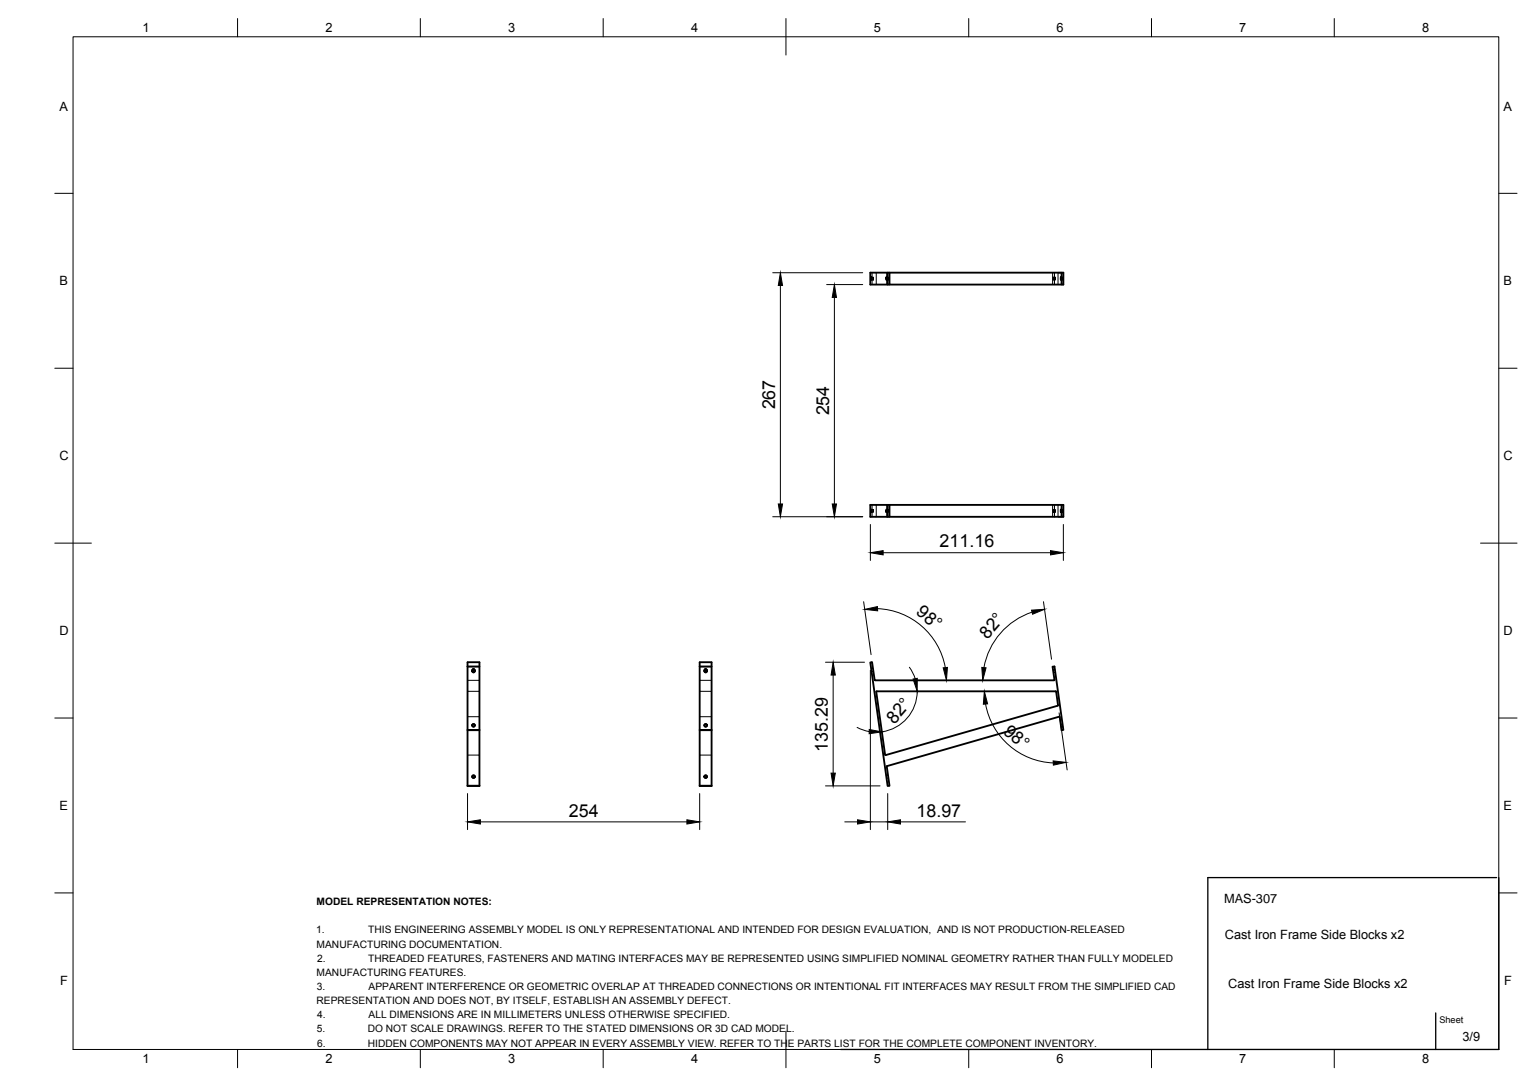
ISO-10303-21;
HEADER;
FILE_DESCRIPTION (('STEP AP214'),
    '1' );
FILE_NAME ('Cast Iron Frame Side Blocks x2.step',
    '2026-10-06T07:34:29',
    ( '' ),
    ( '' ),
    'SwSTEP 2.0',
    'SolidWorks 2025',
    '' );
FILE_SCHEMA (( 'AUTOMOTIVE_DESIGN' ));
ENDSEC;

DATA;
#2=DIRECTION ( 'NONE',  ( 0.000000000000000000, 0.000000000000000000, -1.000000000000000000 ) ) ;
#4=CARTESIAN_POINT ( 'NONE',  ( 177.5000000000000853, 15.47035339324670922, 37.00486596562913633 ) ) ;
#7=CARTESIAN_POINT ( 'NONE',  ( -70.00000000000000000, -201.3058001507315566, -41.45141194869120227 ) ) ;
#12=ORIENTED_EDGE ( 'NONE', *, *, #8305, .F. ) ;
#13=DIRECTION ( 'NONE',  ( 0.000000000000000000, 0.1391731009600660485, -0.9902680687415702510 ) ) ;
#19=ORIENTED_EDGE ( 'NONE', *, *, #12875, .F. ) ;
#22=ORIENTED_EDGE ( 'NONE', *, *, #8785, .F. ) ;
#31=ORIENTED_EDGE ( 'NONE', *, *, #9479, .F. ) ;
#35=LINE ( 'NONE', #4552, #8075 ) ;
#37=DIRECTION ( 'NONE',  ( 0.000000000000000000, 0.000000000000000000, -1.000000000000000000 ) ) ;
#45=CARTESIAN_POINT ( 'NONE',  ( -76.50000000000001421, 15.03993994372673981, 10.05257423913146475 ) ) ;
#48=CARTESIAN_POINT ( 'NONE',  ( 177.5000000000000853, 15.03993994372673804, 24.94742576086838781 ) ) ;
#54=FACE_OUTER_BOUND ( 'NONE', #8334, .T. ) ;
#65=LINE ( 'NONE', #4977, #10142 ) ;
#67=VECTOR ( 'NONE', #9001, 1000.000000000000000 ) ;
#69=EDGE_LOOP ( 'NONE', ( #4641, #9788 ) ) ;
#70=DIRECTION ( 'NONE',  ( -3.965082230804130220E-16, -0.000000000000000000, -1.000000000000000000 ) ) ;
#72=EDGE_CURVE ( 'NONE', #11235, #14746, #6724, .T. ) ;
#73=AXIS2_PLACEMENT_3D ( 'NONE', #11589, #11673, #2027 ) ;
#74=ORIENTED_EDGE ( 'NONE', *, *, #9272, .F. ) ;
#75=FACE_OUTER_BOUND ( 'NONE', #2731, .T. ) ;
#78=VECTOR ( 'NONE', #416, 1000.000000000000000 ) ;
#85=VERTEX_POINT ( 'NONE', #2360 ) ;
#89=ORIENTED_EDGE ( 'NONE', *, *, #715, .T. ) ;
#91=FACE_OUTER_BOUND ( 'NONE', #15309, .T. ) ;
#92=CARTESIAN_POINT ( 'NONE',  ( 178.0000000000000853, 15.03993994372673981, -3.075184203610571654 ) ) ;
#96=ORIENTED_EDGE ( 'NONE', *, *, #2656, .T. ) ;
#98=CARTESIAN_POINT ( 'NONE',  ( 175.9483885134608272, -181.3058001507315566, -51.45141194869120227 ) ) ;
#101=VERTEX_POINT ( 'NONE', #4890 ) ;
#108=VECTOR ( 'NONE', #10524, 1000.000000000000000 ) ;
#115=AXIS2_PLACEMENT_3D ( 'NONE', #5696, #3243, #10590 ) ;
#118=ORIENTED_EDGE ( 'NONE', *, *, #6762, .T. ) ;
#121=ORIENTED_EDGE ( 'NONE', *, *, #6164, .F. ) ;
#122=DIRECTION ( 'NONE',  ( 1.000000000000000000, 0.000000000000000000, 0.000000000000000000 ) ) ;
#128=DIRECTION ( 'NONE',  ( 0.000000000000000000, 0.000000000000000000, -1.000000000000000000 ) ) ;
#129=AXIS2_PLACEMENT_3D ( 'NONE', #758, #2991, #9229 ) ;
#134=ORIENTED_EDGE ( 'NONE', *, *, #1310, .F. ) ;
#138=VERTEX_POINT ( 'NONE', #10733 ) ;
#140=AXIS2_PLACEMENT_3D ( 'NONE', #4727, #9874, #2603 ) ;
#141=CARTESIAN_POINT ( 'NONE',  ( 177.5000000000000853, -179.3058001507315566, -51.45141194869120227 ) ) ;
#144=CARTESIAN_POINT ( 'NONE',  ( 114.0000000000000426, 15.53993994372673981, 7.305634244248866343E-16 ) ) ;
#145=DIRECTION ( 'NONE',  ( -5.518327896226365911E-17, 0.9902680687415714722, -0.1391731009600582769 ) ) ;
#148=EDGE_LOOP ( 'NONE', ( #966, #9881, #15338, #13043 ) ) ;
#150=CARTESIAN_POINT ( 'NONE',  ( 190.5000000000000568, -181.3058001507315566, 84.88378295107885663 ) ) ;
#151=ORIENTED_EDGE ( 'NONE', *, *, #11944, .F. ) ;
#154=ORIENTED_EDGE ( 'NONE', *, *, #12875, .T. ) ;
#160=DIRECTION ( 'NONE',  ( 0.000000000000000000, 0.9902680687415712502, 0.1391731009600584990 ) ) ;
#161=DIRECTION ( 'NONE',  ( 0.000000000000000000, 0.000000000000000000, -1.000000000000000000 ) ) ;
#164=EDGE_CURVE ( 'NONE', #1358, #7203, #12629, .T. ) ;
#165=LINE ( 'NONE', #5013, #3777 ) ;
#168=CARTESIAN_POINT ( 'NONE',  ( -64.00000000000002842, 15.53993994372673981, -3.075184203610571654 ) ) ;
#171=CARTESIAN_POINT ( 'NONE',  ( -63.50000000000002842, 15.03993994372673981, -3.075184203610571654 ) ) ;
#172=ORIENTED_EDGE ( 'NONE', *, *, #9722, .T. ) ;
#176=VERTEX_POINT ( 'NONE', #14424 ) ;
#177=AXIS2_PLACEMENT_3D ( 'NONE', #9070, #13874, #12756 ) ;
#180=( GEOMETRIC_REPRESENTATION_CONTEXT ( 3 ) GLOBAL_UNCERTAINTY_ASSIGNED_CONTEXT ( ( #8186 ) ) GLOBAL_UNIT_ASSIGNED_CONTEXT ( ( #3150, #4481, #1954 ) ) REPRESENTATION_CONTEXT ( 'NONE', 'WORKASPACE' ) );
#182=TOROIDAL_SURFACE ( 'NONE', #1206, 1.000000000000000000, 0.5000000000000000000 ) ;
#185=AXIS2_PLACEMENT_3D ( 'NONE', #1249, #10903, #14351 ) ;
#187=DIRECTION ( 'NONE',  ( 0.000000000000000000, 0.000000000000000000, 1.000000000000000000 ) ) ;
#190=ADVANCED_FACE ( 'NONE', ( #12144 ), #4855, .T. ) ;
#194=LINE ( 'NONE', #8457, #6371 ) ;
#196=DIRECTION ( 'NONE',  ( 0.000000000000000000, 0.000000000000000000, 1.000000000000000000 ) ) ;
#200=VECTOR ( 'NONE', #3620, 1000.000000000000000 ) ;
#201=EDGE_LOOP ( 'NONE', ( #1693, #11095, #14591, #7867 ) ) ;
#202=AXIS2_PLACEMENT_3D ( 'NONE', #6427, #5227, #1671 ) ;
#203=EDGE_CURVE ( 'NONE', #12014, #13507, #9648, .T. ) ;
#213=CIRCLE ( 'NONE', #730, 1.000000000000000888 ) ;
#216=CARTESIAN_POINT ( 'NONE',  ( -61.94838851346079167, -178.8058001507315566, 52.69066787724494816 ) ) ;
#217=CARTESIAN_POINT ( 'NONE',  ( -76.00000000000001421, 15.53993994372674159, 9.617930870223352358 ) ) ;
#225=EDGE_CURVE ( 'NONE', #176, #7789, #1243, .T. ) ;
#227=VERTEX_POINT ( 'NONE', #12067 ) ;
#228=LINE ( 'NONE', #150, #2384 ) ;
#234=VERTEX_POINT ( 'NONE', #13400 ) ;
#235=VERTEX_POINT ( 'NONE', #8458 ) ;
#238=VECTOR ( 'NONE', #1875, 1000.000000000000000 ) ;
#239=ORIENTED_EDGE ( 'NONE', *, *, #3705, .T. ) ;
#241=CARTESIAN_POINT ( 'NONE',  ( 190.0000000000000568, -179.3058001507315282, -29.88378295107906268 ) ) ;
#242=FACE_OUTER_BOUND ( 'NONE', #9642, .T. ) ;
#245=EDGE_CURVE ( 'NONE', #3324, #6496, #6158, .T. ) ;
#246=AXIS2_PLACEMENT_3D ( 'NONE', #10758, #10919, #3716 ) ;
#247=CIRCLE ( 'NONE', #14631, 0.5000000000000069944 ) ;
#248=( LENGTH_UNIT ( ) NAMED_UNIT ( * ) SI_UNIT ( .MILLI., .METRE. ) );
#251=DIRECTION ( 'NONE',  ( 0.000000000000000000, 6.938893903907227145E-17, -1.000000000000000000 ) ) ;
#260=EDGE_LOOP ( 'NONE', ( #8120, #14477, #13087, #8621 ) ) ;
#264=CARTESIAN_POINT ( 'NONE',  ( 0.000000000000000000, 17.53993994372673981, 8.693413025030312018E-16 ) ) ;
#268=AXIS2_PLACEMENT_3D ( 'NONE', #5608, #7835, #11451 ) ;
#274=FACE_BOUND ( 'NONE', #5485, .T. ) ;
#279=ORIENTED_EDGE ( 'NONE', *, *, #13409, .F. ) ;
#283=CARTESIAN_POINT ( 'NONE',  ( -64.00000000000002842, -179.3058001507315566, 52.76585208085545275 ) ) ;
#285=DIRECTION ( 'NONE',  ( 1.000000000000000000, -2.751328491981765035E-32, 3.965082230804130220E-16 ) ) ;
#290=ORIENTED_EDGE ( 'NONE', *, *, #8264, .F. ) ;
#296=LINE ( 'NONE', #14821, #5534 ) ;
#297=VECTOR ( 'NONE', #7988, 1000.000000000000000 ) ;
#301=DIRECTION ( 'NONE',  ( -0.000000000000000000, 6.938893903907222067E-15, -1.000000000000000000 ) ) ;
#310=EDGE_CURVE ( 'NONE', #12060, #3478, #2754, .T. ) ;
#313=CARTESIAN_POINT ( 'NONE',  ( 178.0000000000000853, -179.3058001507315566, 84.88378295107887084 ) ) ;
#322=CARTESIAN_POINT ( 'NONE',  ( -64.00000000000002842, -178.8058001507315566, -17.19066787724516843 ) ) ;
#323=CARTESIAN_POINT ( 'NONE',  ( 184.0000000000000568, -179.3058001507315566, 76.45141194869098911 ) ) ;
#331=DIRECTION ( 'NONE',  ( 0.000000000000000000, -0.1391731009600591096, 0.9902680687415711391 ) ) ;
#332=EDGE_LOOP ( 'NONE', ( #12624, #8209, #7735, #9718 ) ) ;
#335=EDGE_CURVE ( 'NONE', #2939, #10298, #8373, .T. ) ;
#336=AXIS2_PLACEMENT_3D ( 'NONE', #14411, #13144, #5897 ) ;
#339=ORIENTED_EDGE ( 'NONE', *, *, #2372, .F. ) ;
#341=CYLINDRICAL_SURFACE ( 'NONE', #1669, 0.5000000000000004441 ) ;
#345=CARTESIAN_POINT ( 'NONE',  ( 190.0000000000001137, -179.3058001507315566, 84.88378295107887084 ) ) ;
#347=CARTESIAN_POINT ( 'NONE',  ( -76.50000000000001421, 15.53993994372673981, -17.50000000000002487 ) ) ;
#351=ORIENTED_EDGE ( 'NONE', *, *, #9722, .F. ) ;
#360=ORIENTED_EDGE ( 'NONE', *, *, #11900, .T. ) ;
#361=AXIS2_PLACEMENT_3D ( 'NONE', #5638, #4281, #10375 ) ;
#364=EDGE_CURVE ( 'NONE', #10667, #14434, #6613, .T. ) ;
#365=ADVANCED_FACE ( 'NONE', ( #3595 ), #14635, .F. ) ;
#375=CARTESIAN_POINT ( 'NONE',  ( 178.0000000000000853, -178.8058001507315566, 52.69066787724494816 ) ) ;
#377=VECTOR ( 'NONE', #4213, 1000.000000000000000 ) ;
#383=CARTESIAN_POINT ( 'NONE',  ( 177.5000000000000853, -178.8058001507315566, 52.19066787724494816 ) ) ;
#384=DIRECTION ( 'NONE',  ( -0.000000000000000000, -0.000000000000000000, 1.000000000000000000 ) ) ;
#387=AXIS2_PLACEMENT_3D ( 'NONE', #2185, #5898, #3681 ) ;
#389=ORIENTED_EDGE ( 'NONE', *, *, #3413, .F. ) ;
#390=ORIENTED_EDGE ( 'NONE', *, *, #8566, .T. ) ;
#396=DIRECTION ( 'NONE',  ( 0.000000000000000000, 0.000000000000000000, -1.000000000000000000 ) ) ;
#398=DIRECTION ( 'NONE',  ( -1.000000000000000000, -0.000000000000000000, -0.000000000000000000 ) ) ;
#399=CIRCLE ( 'NONE', #3701, 1.000000000000000888 ) ;
#400=CARTESIAN_POINT ( 'NONE',  ( -76.50000000000004263, 16.03993994372673981, 24.94742576086838781 ) ) ;
#403=ORIENTED_EDGE ( 'NONE', *, *, #203, .F. ) ;
#416=DIRECTION ( 'NONE',  ( -0.000000000000000000, 1.000000000000000000, -0.000000000000000000 ) ) ;
#417=ADVANCED_FACE ( 'NONE', ( #6046 ), #9121, .T. ) ;
#423=CARTESIAN_POINT ( 'NONE',  ( 178.0000000000000853, 15.03993994372673804, 24.94742576086838781 ) ) ;
#424=ORIENTED_EDGE ( 'NONE', *, *, #5483, .F. ) ;
#426=CIRCLE ( 'NONE', #15310, 0.5000000000000004441 ) ;
#427=VERTEX_POINT ( 'NONE', #7398 ) ;
#431=AXIS2_PLACEMENT_3D ( 'NONE', #11990, #8295, #10275 ) ;
#433=CARTESIAN_POINT ( 'NONE',  ( -63.50000000000002842, -178.8753867012115961, -29.82329228561640022 ) ) ;
#436=EDGE_CURVE ( 'NONE', #7205, #8201, #10784, .T. ) ;
#445=EDGE_CURVE ( 'NONE', #10124, #3324, #12383, .T. ) ;
#450=ORIENTED_EDGE ( 'NONE', *, *, #1874, .F. ) ;
#455=EDGE_CURVE ( 'NONE', #6271, #3832, #8131, .T. ) ;
#459=ORIENTED_EDGE ( 'NONE', *, *, #5935, .T. ) ;
#460=AXIS2_PLACEMENT_3D ( 'NONE', #7389, #8262, #9589 ) ;
#461=DIRECTION ( 'NONE',  ( -1.000000000000000000, 0.000000000000000000, 0.000000000000000000 ) ) ;
#463=CARTESIAN_POINT ( 'NONE',  ( 175.9483885134608272, -181.3058001507315566, 84.88378295107885663 ) ) ;
#465=CARTESIAN_POINT ( 'NONE',  ( 177.5000000000000853, 17.53993994372673626, 52.49999999999997868 ) ) ;
#466=EDGE_LOOP ( 'NONE', ( #4763, #4256, #4464, #11811 ) ) ;
#468=LINE ( 'NONE', #553, #2479 ) ;
#474=VECTOR ( 'NONE', #4202, 1000.000000000000000 ) ;
#476=FACE_OUTER_BOUND ( 'NONE', #10606, .T. ) ;
#477=CARTESIAN_POINT ( 'NONE',  ( -76.00000000000004263, -178.6666270497714777, 53.18093594598651919 ) ) ;
#478=VECTOR ( 'NONE', #15395, 1000.000000000000000 ) ;
#480=VECTOR ( 'NONE', #1184, 1000.000000000000000 ) ;
#481=ORIENTED_EDGE ( 'NONE', *, *, #8412, .F. ) ;
#484=AXIS2_PLACEMENT_3D ( 'NONE', #5944, #4676, #14380 ) ;
#486=DIRECTION ( 'NONE',  ( -1.000000000000000000, 0.000000000000000000, 0.000000000000000000 ) ) ;
#495=AXIS2_PLACEMENT_3D ( 'NONE', #10525, #9661, #9579 ) ;
#496=CIRCLE ( 'NONE', #12110, 0.5000000000000000000 ) ;
#501=CARTESIAN_POINT ( 'NONE',  ( -76.00000000000001421, -179.8058001507315566, -17.50000000000002487 ) ) ;
#502=CIRCLE ( 'NONE', #9361, 1.000000000000000888 ) ;
#510=CARTESIAN_POINT ( 'NONE',  ( 190.0000000000000853, 15.03993994372673804, 38.07518420361041933 ) ) ;
#515=LINE ( 'NONE', #433, #1175 ) ;
#520=ORIENTED_EDGE ( 'NONE', *, *, #10311, .F. ) ;
#524=CARTESIAN_POINT ( 'NONE',  ( -61.94838851346079167, -179.3058001507315566, 84.88378295107887084 ) ) ;
#526=CARTESIAN_POINT ( 'NONE',  ( -64.00000000000002842, 15.10952649420676863, 9.557440204760682789 ) ) ;
#530=ORIENTED_EDGE ( 'NONE', *, *, #7219, .T. ) ;
#532=CARTESIAN_POINT ( 'NONE',  ( -76.50000000000004263, 16.03993994372673626, 38.07518420361041933 ) ) ;
#533=TOROIDAL_SURFACE ( 'NONE', #1054, 1.000000000000000000, 0.5000000000000000000 ) ;
#534=EDGE_CURVE ( 'NONE', #12538, #8345, #9996, .T. ) ;
#537=EDGE_CURVE ( 'NONE', #9039, #10463, #3828, .T. ) ;
#541=ORIENTED_EDGE ( 'NONE', *, *, #1567, .F. ) ;
#549=EDGE_CURVE ( 'NONE', #10298, #12812, #1611, .T. ) ;
#552=VERTEX_POINT ( 'NONE', #6443 ) ;
#553=CARTESIAN_POINT ( 'NONE',  ( -64.00000000000002842, 15.53993994372674159, -17.50000000000002487 ) ) ;
#554=CARTESIAN_POINT ( 'NONE',  ( 114.0000000000000426, 15.03993994372673804, 38.07518420361041933 ) ) ;
#558=DIRECTION ( 'NONE',  ( 0.000000000000000000, 1.000000000000000000, 6.938893903907227145E-17 ) ) ;
#559=DIRECTION ( 'NONE',  ( -5.518327896226364679E-17, 0.9902680687415713612, -0.1391731009600582492 ) ) ;
#561=AXIS2_PLACEMENT_3D ( 'NONE', #1268, #5934, #15618 ) ;
#564=PRODUCT_DEFINITION_SHAPE ( 'NONE', 'NONE',  #12586 ) ;
#567=EDGE_CURVE ( 'NONE', #8004, #6496, #10133, .T. ) ;
#568=EDGE_LOOP ( 'NONE', ( #1581, #6786, #11329, #3119, #5472 ) ) ;
#571=DIRECTION ( 'NONE',  ( -1.000000000000000000, -2.751328491981765035E-32, 3.965082230804130220E-16 ) ) ;
#572=ORIENTED_EDGE ( 'NONE', *, *, #10492, .T. ) ;
#578=AXIS2_PLACEMENT_3D ( 'NONE', #12146, #8381, #196 ) ;
#581=LINE ( 'NONE', #14871, #3041 ) ;
#582=CARTESIAN_POINT ( 'NONE',  ( -64.00000000000002842, 16.03993994372673626, 52.49999999999997868 ) ) ;
#583=ORIENTED_EDGE ( 'NONE', *, *, #567, .T. ) ;
#584=DIRECTION ( 'NONE',  ( 1.000000000000000000, 2.751328491981765035E-32, -3.965082230804130220E-16 ) ) ;
#585=CIRCLE ( 'NONE', #7676, 0.4999999999999996114 ) ;
#587=DIRECTION ( 'NONE',  ( 3.965082230804130220E-16, 0.000000000000000000, -1.000000000000000000 ) ) ;
#590=LINE ( 'NONE', #14959, #5579 ) ;
#592=VERTEX_POINT ( 'NONE', #2722 ) ;
#602=CARTESIAN_POINT ( 'NONE',  ( -70.00000000000000000, -179.3058001507315566, 77.95141194869098911 ) ) ;
#607=ADVANCED_FACE ( 'NONE', ( #2807 ), #5240, .T. ) ;
#609=CARTESIAN_POINT ( 'NONE',  ( 190.0000000000000568, 16.03993994372673981, -17.50000000000002487 ) ) ;
#610=EDGE_LOOP ( 'NONE', ( #2494, #13099, #11658, #12141 ) ) ;
#612=ORIENTED_EDGE ( 'NONE', *, *, #2131, .T. ) ;
#615=ORIENTED_EDGE ( 'NONE', *, *, #12398, .F. ) ;
#616=DIRECTION ( 'NONE',  ( 0.000000000000000000, 0.000000000000000000, 1.000000000000000000 ) ) ;
#618=VECTOR ( 'NONE', #13285, 1000.000000000000114 ) ;
#619=DIRECTION ( 'NONE',  ( 1.000000000000000000, 0.000000000000000000, 0.000000000000000000 ) ) ;
#620=VERTEX_POINT ( 'NONE', #1173 ) ;
#628=CARTESIAN_POINT ( 'NONE',  ( -76.50000000000001421, -179.8058001507315566, -30.31842631998718574 ) ) ;
#632=ORIENTED_EDGE ( 'NONE', *, *, #3155, .T. ) ;
#635=CARTESIAN_POINT ( 'NONE',  ( 190.0000000000000853, -178.9449732516916072, 64.32815825124538378 ) ) ;
#636=ORIENTED_EDGE ( 'NONE', *, *, #225, .T. ) ;
#640=CARTESIAN_POINT ( 'NONE',  ( -76.00000000000001421, -178.7362136002515172, -17.68580191161595394 ) ) ;
#648=DIRECTION ( 'NONE',  ( 0.000000000000000000, 0.000000000000000000, -1.000000000000000000 ) ) ;
#652=VERTEX_POINT ( 'NONE', #11928 ) ;
#657=EDGE_CURVE ( 'NONE', #11157, #14585, #9638, .T. ) ;
#658=CARTESIAN_POINT ( 'NONE',  ( 190.5000000000000568, -179.2362136002515172, -18.26098611522645498 ) ) ;
#660=CARTESIAN_POINT ( 'NONE',  ( 184.0000000000000568, -201.3058001507315566, 76.45141194869098911 ) ) ;
#664=ORIENTED_EDGE ( 'NONE', *, *, #6908, .T. ) ;
#674=DIRECTION ( 'NONE',  ( 3.965082230804130220E-16, 0.000000000000000000, -1.000000000000000000 ) ) ;
#676=ADVANCED_FACE ( 'NONE', ( #7123 ), #8237, .T. ) ;
#682=ORIENTED_EDGE ( 'NONE', *, *, #14233, .T. ) ;
#683=AXIS2_PLACEMENT_3D ( 'NONE', #8224, #1001, #14265 ) ;
#686=FACE_OUTER_BOUND ( 'NONE', #769, .T. ) ;
#689=DIRECTION ( 'NONE',  ( 1.000000000000000000, 0.000000000000000000, 0.000000000000000000 ) ) ;
#691=ADVANCED_FACE ( 'NONE', ( #3556 ), #4497, .F. ) ;
#695=AXIS2_PLACEMENT_3D ( 'NONE', #4147, #10396, #5501 ) ;
#698=ORIENTED_EDGE ( 'NONE', *, *, #5084, .T. ) ;
#699=FACE_BOUND ( 'NONE', #1042, .T. ) ;
#703=CARTESIAN_POINT ( 'NONE',  ( 190.5000000000000568, -179.8058001507315566, -17.19066787724516843 ) ) ;
#707=VECTOR ( 'NONE', #4697, 1000.000000000000000 ) ;
#708=EDGE_LOOP ( 'NONE', ( #6506, #5405, #10280, #13729 ) ) ;
#710=DIRECTION ( 'NONE',  ( 1.000000000000000000, -2.751328491981765035E-32, 3.965082230804130220E-16 ) ) ;
#714=EDGE_CURVE ( 'NONE', #5220, #7650, #15299, .T. ) ;
#715=EDGE_CURVE ( 'NONE', #10772, #8234, #3323, .T. ) ;
#718=AXIS2_PLACEMENT_3D ( 'NONE', #1049, #5716, #8108 ) ;
#719=LINE ( 'NONE', #10143, #474 ) ;
#720=VERTEX_POINT ( 'NONE', #9959 ) ;
#726=UNCERTAINTY_MEASURE_WITH_UNIT (LENGTH_MEASURE( 1.000000000000000082E-05 ), #3698, 'distance_accuracy_value', 'NONE');
#729=EDGE_LOOP ( 'NONE', ( #13768, #13485, #6754, #10532 ) ) ;
#730=AXIS2_PLACEMENT_3D ( 'NONE', #1202, #9673, #13125 ) ;
#731=EDGE_CURVE ( 'NONE', #11157, #8697, #65, .T. ) ;
#739=ORIENTED_EDGE ( 'NONE', *, *, #8236, .F. ) ;
#740=AXIS2_PLACEMENT_3D ( 'NONE', #3109, #8013, #15241 ) ;
#745=ORIENTED_EDGE ( 'NONE', *, *, #9421, .T. ) ;
#746=LINE ( 'NONE', #15426, #3814 ) ;
#758=CARTESIAN_POINT ( 'NONE',  ( -64.00000000000002842, -178.8058001507315566, -17.19066787724516843 ) ) ;
#761=DIRECTION ( 'NONE',  ( 0.000000000000000000, -6.938893903907222067E-15, 1.000000000000000000 ) ) ;
#763=DIRECTION ( 'NONE',  ( -1.000000000000000000, -0.000000000000000000, -0.000000000000000000 ) ) ;
#764=DIRECTION ( 'NONE',  ( 0.000000000000000000, 0.000000000000000000, -1.000000000000000000 ) ) ;
#767=ORIENTED_EDGE ( 'NONE', *, *, #14509, .T. ) ;
#769=EDGE_LOOP ( 'NONE', ( #6172, #937, #13033, #15405 ) ) ;
#777=CARTESIAN_POINT ( 'NONE',  ( 178.0000000000000853, -178.7362136002515172, 52.68580191161573367 ) ) ;
#779=ORIENTED_EDGE ( 'NONE', *, *, #13958, .F. ) ;
#781=CARTESIAN_POINT ( 'NONE',  ( -64.00000000000002842, -178.8058001507315566, 52.19066787724494816 ) ) ;
#783=CARTESIAN_POINT ( 'NONE',  ( 178.0000000000000853, -178.7362136002515172, -17.68580191161595394 ) ) ;
#787=EDGE_LOOP ( 'NONE', ( #6983, #4310, #14077, #11881 ) ) ;
#789=AXIS2_PLACEMENT_3D ( 'NONE', #609, #10339, #13796 ) ;
#793=ORIENTED_EDGE ( 'NONE', *, *, #9332, .T. ) ;
#796=DIRECTION ( 'NONE',  ( 0.000000000000000000, -1.000000000000000000, 0.000000000000000000 ) ) ;
#797=CARTESIAN_POINT ( 'NONE',  ( 184.0000000000000568, 15.53993994372673981, -13.99999999999999112 ) ) ;
#798=CARTESIAN_POINT ( 'NONE',  ( -64.00000000000002842, -178.8058001507315566, -17.19066787724516843 ) ) ;
#800=AXIS2_PLACEMENT_3D ( 'NONE', #12219, #14347, #9547 ) ;
#801=DIRECTION ( 'NONE',  ( 0.000000000000000000, -1.000000000000000000, -4.956352788505160310E-17 ) ) ;
#802=ORIENTED_EDGE ( 'NONE', *, *, #15381, .T. ) ;
#804=EDGE_CURVE ( 'NONE', #3126, #11344, #6868, .T. ) ;
#806=DIRECTION ( 'NONE',  ( -0.000000000000000000, -0.9902680687415713612, 0.1391731009600582492 ) ) ;
#814=LINE ( 'NONE', #11569, #14126 ) ;
#815=VERTEX_POINT ( 'NONE', #2530 ) ;
#816=DIRECTION ( 'NONE',  ( 0.000000000000000000, 0.000000000000000000, -1.000000000000000000 ) ) ;
#818=ORIENTED_EDGE ( 'NONE', *, *, #8671, .T. ) ;
#823=EDGE_CURVE ( 'NONE', #235, #10036, #14913, .T. ) ;
#827=PRODUCT ( 'Cast Iron Frame Side Blocks x2', 'Cast Iron Frame Side Blocks x2', '', ( #6581 ) ) ;
#830=VERTEX_POINT ( 'NONE', #4242 ) ;
#831=VERTEX_POINT ( 'NONE', #526 ) ;
#832=DIRECTION ( 'NONE',  ( -0.000000000000000000, -1.000000000000000000, -0.000000000000000000 ) ) ;
#833=PLANE ( 'NONE',  #7276 ) ;
#838=DIRECTION ( 'NONE',  ( 1.000000000000000000, 0.000000000000000000, 0.000000000000000000 ) ) ;
#840=AXIS2_PLACEMENT_3D ( 'NONE', #12273, #3526, #37 ) ;
#854=DIRECTION ( 'NONE',  ( 1.000000000000000000, 2.751328491981765035E-32, -3.965082230804130220E-16 ) ) ;
#862=ORIENTED_EDGE ( 'NONE', *, *, #15336, .F. ) ;
#869=ORIENTED_EDGE ( 'NONE', *, *, #13066, .F. ) ;
#877=CARTESIAN_POINT ( 'NONE',  ( -61.94838851346079167, -179.3058001507315566, 84.88378295107887084 ) ) ;
#878=VECTOR ( 'NONE', #7399, 1000.000000000000000 ) ;
#879=DIRECTION ( 'NONE',  ( -0.000000000000000000, 0.000000000000000000, -1.000000000000000000 ) ) ;
#881=ADVANCED_FACE ( 'NONE', ( #4803 ), #11148, .T. ) ;
#884=CARTESIAN_POINT ( 'NONE',  ( 184.0000000000000568, 15.53993994372673626, 47.49999999999997868 ) ) ;
#885=ORIENTED_EDGE ( 'NONE', *, *, #8221, .F. ) ;
#888=EDGE_LOOP ( 'NONE', ( #12867, #4817, #14342, #1072 ) ) ;
#890=TOROIDAL_SURFACE ( 'NONE', #14004, 1.000000000000000000, 0.5000000000000000000 ) ;
#892=DIRECTION ( 'NONE',  ( 1.000000000000000000, -2.751328491981765035E-32, 3.965082230804130220E-16 ) ) ;
#893=AXIS2_PLACEMENT_3D ( 'NONE', #8643, #9908, #8719 ) ;
#894=DIRECTION ( 'NONE',  ( 3.965082230804130220E-16, 1.090924371466202084E-47, 1.000000000000000000 ) ) ;
#896=ORIENTED_EDGE ( 'NONE', *, *, #6653, .T. ) ;
#904=AXIS2_PLACEMENT_3D ( 'NONE', #11636, #9194, #4125 ) ;
#915=EDGE_CURVE ( 'NONE', #3320, #10463, #3385, .T. ) ;
#918=CARTESIAN_POINT ( 'NONE',  ( 190.0000000000000568, 15.53993994372673981, -2.500000000000071054 ) ) ;
#919=CIRCLE ( 'NONE', #9009, 1.000000000000000888 ) ;
#921=EDGE_CURVE ( 'NONE', #12187, #12589, #5102, .T. ) ;
#923=CARTESIAN_POINT ( 'NONE',  ( -76.00000000000001421, 16.03993994372673981, -7.458121719691109004E-14 ) ) ;
#928=PLANE ( 'NONE',  #9563 ) ;
#932=FILL_AREA_STYLE ('',( #8154 ) ) ;
#934=ADVANCED_FACE ( 'NONE', ( #11911 ), #13001, .T. ) ;
#937=ORIENTED_EDGE ( 'NONE', *, *, #4830, .T. ) ;
#939=CARTESIAN_POINT ( 'NONE',  ( -63.50000000000002842, -179.8058001507315566, -51.45141194869119516 ) ) ;
#943=PLANE ( 'NONE',  #13809 ) ;
#944=VERTEX_POINT ( 'NONE', #5832 ) ;
#945=ORIENTED_EDGE ( 'NONE', *, *, #7328, .T. ) ;
#946=DIRECTION ( 'NONE',  ( 0.000000000000000000, 0.000000000000000000, 1.000000000000000000 ) ) ;
#947=LINE ( 'NONE', #141, #14146 ) ;
#949=ORIENTED_EDGE ( 'NONE', *, *, #2798, .T. ) ;
#951=DIRECTION ( 'NONE',  ( -2.897122145519000304E-15, 0.9902680687415702510, 0.1391731009600660485 ) ) ;
#952=CIRCLE ( 'NONE', #13851, 0.5000000000000004441 ) ;
#961=DIRECTION ( 'NONE',  ( 0.000000000000000000, 0.000000000000000000, 1.000000000000000000 ) ) ;
#962=PLANE ( 'NONE',  #6800 ) ;
#966=ORIENTED_EDGE ( 'NONE', *, *, #12260, .T. ) ;
#980=LINE ( 'NONE', #14245, #1723 ) ;
#985=ORIENTED_EDGE ( 'NONE', *, *, #11407, .T. ) ;
#986=EDGE_LOOP ( 'NONE', ( #15497, #15442, #9179, #14463 ) ) ;
#987=FACE_OUTER_BOUND ( 'NONE', #2580, .T. ) ;
#989=EDGE_CURVE ( 'NONE', #4028, #7962, #7888, .T. ) ;
#994=AXIS2_PLACEMENT_3D ( 'NONE', #12797, #10367, #1984 ) ;
#1001=DIRECTION ( 'NONE',  ( -1.000000000000000000, 0.000000000000000000, 0.000000000000000000 ) ) ;
#1002=CIRCLE ( 'NONE', #10862, 1.499999999999994449 ) ;
#1003=DIRECTION ( 'NONE',  ( 0.000000000000000000, 0.1391731009600592484, 0.9902680687415712502 ) ) ;
#1004=ORIENTED_EDGE ( 'NONE', *, *, #2372, .T. ) ;
#1008=CARTESIAN_POINT ( 'NONE',  ( -63.50000000000002842, -179.8058001507315566, 84.88378295107887084 ) ) ;
#1010=DIRECTION ( 'NONE',  ( -1.000000000000000000, 0.000000000000000000, 0.000000000000000000 ) ) ;
#1020=ORIENTED_EDGE ( 'NONE', *, *, #14970, .T. ) ;
#1030=ORIENTED_EDGE ( 'NONE', *, *, #12016, .T. ) ;
#1033=LINE ( 'NONE', #4508, #9633 ) ;
#1034=AXIS2_PLACEMENT_3D ( 'NONE', #635, #3025, #4190 ) ;
#1035=ORIENTED_EDGE ( 'NONE', *, *, #1489, .T. ) ;
#1041=ADVANCED_FACE ( 'NONE', ( #2431 ), #2744, .F. ) ;
#1042=EDGE_LOOP ( 'NONE', ( #11606, #15270 ) ) ;
#1049=CARTESIAN_POINT ( 'NONE',  ( -76.00000000000001421, 15.03993994372673981, -3.075184203610571654 ) ) ;
#1054=AXIS2_PLACEMENT_3D ( 'NONE', #1853, #3198, #15183 ) ;
#1055=CARTESIAN_POINT ( 'NONE',  ( 190.5000000000000568, 15.03993994372673981, -3.075184203610571654 ) ) ;
#1058=DIRECTION ( 'NONE',  ( 1.000000000000000000, 0.000000000000000000, 0.000000000000000000 ) ) ;
#1060=ORIENTED_EDGE ( 'NONE', *, *, #7722, .T. ) ;
#1062=CARTESIAN_POINT ( 'NONE',  ( 178.0000000000000853, -178.8058001507315566, 65.31842631998698323 ) ) ;
#1072=ORIENTED_EDGE ( 'NONE', *, *, #11053, .F. ) ;
#1077=EDGE_CURVE ( 'NONE', #10971, #14401, #8747, .T. ) ;
#1080=VECTOR ( 'NONE', #3010, 1000.000000000000000 ) ;
#1099=AXIS2_PLACEMENT_3D ( 'NONE', #524, #761, #9079 ) ;
#1101=CARTESIAN_POINT ( 'NONE',  ( 190.0000000000000568, 13.40307322461932493, -2.295403246091865412 ) ) ;
#1103=CARTESIAN_POINT ( 'NONE',  ( 175.9483885134608272, 15.03993994372673981, -3.075184203610571654 ) ) ;
#1106=EDGE_LOOP ( 'NONE', ( #4528, #9454, #14687, #11346 ) ) ;
#1107=ORIENTED_EDGE ( 'NONE', *, *, #3537, .T. ) ;
#1112=AXIS2_PLACEMENT_3D ( 'NONE', #7296, #5521, #12474 ) ;
#1116=ADVANCED_FACE ( 'NONE', ( #8520, #13469, #274 ), #7343, .F. ) ;
#1119=DIRECTION ( 'NONE',  ( 3.965082230804130220E-16, 0.000000000000000000, 1.000000000000000000 ) ) ;
#1120=ORIENTED_EDGE ( 'NONE', *, *, #3798, .F. ) ;
#1124=DIRECTION ( 'NONE',  ( 0.000000000000000000, 1.000000000000000000, 6.938893903907227145E-17 ) ) ;
#1132=DIRECTION ( 'NONE',  ( 1.000000000000000000, 0.000000000000000000, 0.000000000000000000 ) ) ;
#1135=FACE_OUTER_BOUND ( 'NONE', #5191, .T. ) ;
#1137=VERTEX_POINT ( 'NONE', #9938 ) ;
#1149=CARTESIAN_POINT ( 'NONE',  ( -76.00000000000001421, -179.8058001507315566, -17.19066787724516843 ) ) ;
#1154=DIRECTION ( 'NONE',  ( 0.000000000000000000, 1.000000000000000000, 0.000000000000000000 ) ) ;
#1156=CARTESIAN_POINT ( 'NONE',  ( 178.0000000000000853, 15.03993994372673804, 38.07518420361041933 ) ) ;
#1157=CARTESIAN_POINT ( 'NONE',  ( -63.50000000000002842, 14.97035339324670744, 37.58005016923963382 ) ) ;
#1160=DIRECTION ( 'NONE',  ( 0.000000000000000000, 0.000000000000000000, 1.000000000000000000 ) ) ;
#1165=CARTESIAN_POINT ( 'NONE',  ( 175.9483885134608272, 15.03993994372673981, -2.575184203610571654 ) ) ;
#1170=ORIENTED_EDGE ( 'NONE', *, *, #14936, .F. ) ;
#1173=CARTESIAN_POINT ( 'NONE',  ( 178.0000000000000853, -178.8058001507315566, -17.69066787724516843 ) ) ;
#1175=VECTOR ( 'NONE', #10098, 1000.000000000000000 ) ;
#1178=VERTEX_POINT ( 'NONE', #10894 ) ;
#1181=EDGE_CURVE ( 'NONE', #13859, #5228, #502, .T. ) ;
#1184=DIRECTION ( 'NONE',  ( 0.000000000000000000, 1.000000000000000000, 0.000000000000000000 ) ) ;
#1187=EDGE_CURVE ( 'NONE', #227, #1631, #1934, .T. ) ;
#1188=CARTESIAN_POINT ( 'NONE',  ( -63.50000000000002842, 17.53993994372673626, 52.49999999999997868 ) ) ;
#1190=CYLINDRICAL_SURFACE ( 'NONE', #4296, 1.499999999999994449 ) ;
#1193=ORIENTED_EDGE ( 'NONE', *, *, #2572, .F. ) ;
#1198=EDGE_CURVE ( 'NONE', #5867, #10763, #5282, .T. ) ;
#1202=CARTESIAN_POINT ( 'NONE',  ( 190.5000000000000853, 15.03993994372673804, 38.07518420361041933 ) ) ;
#1203=AXIS2_PLACEMENT_3D ( 'NONE', #3408, #15232, #11541 ) ;
#1206=AXIS2_PLACEMENT_3D ( 'NONE', #7566, #6150, #9937 ) ;
#1221=CIRCLE ( 'NONE', #8799, 1.499999999999994449 ) ;
#1225=AXIS2_PLACEMENT_3D ( 'NONE', #14550, #2571, #8505 ) ;
#1229=CARTESIAN_POINT ( 'NONE',  ( 178.0000000000000853, 15.53993994372673981, -3.075184203610571654 ) ) ;
#1230=CIRCLE ( 'NONE', #10074, 0.5000000000000001110 ) ;
#1233=VECTOR ( 'NONE', #806, 1000.000000000000114 ) ;
#1235=CARTESIAN_POINT ( 'NONE',  ( -76.50000000000001421, 16.03993994372673981, 9.617930870223348805 ) ) ;
#1236=DIRECTION ( 'NONE',  ( 0.000000000000000000, 4.956352788505162775E-17, -1.000000000000000000 ) ) ;
#1237=ORIENTED_EDGE ( 'NONE', *, *, #7297, .T. ) ;
#1238=EDGE_LOOP ( 'NONE', ( #9544, #15230, #13995, #7422 ) ) ;
#1240=DIRECTION ( 'NONE',  ( -1.000000000000000000, 0.000000000000000000, 0.000000000000000000 ) ) ;
#1241=CARTESIAN_POINT ( 'NONE',  ( -64.00000000000002842, 14.97035339324670922, -2.580050169239785696 ) ) ;
#1243=LINE ( 'NONE', #3465, #6640 ) ;
#1244=CIRCLE ( 'NONE', #10080, 1.499999999999997780 ) ;
#1249=CARTESIAN_POINT ( 'NONE',  ( -61.94838851346079167, -178.8058001507315566, 52.19066787724494816 ) ) ;
#1254=ORIENTED_EDGE ( 'NONE', *, *, #14681, .F. ) ;
#1262=ORIENTED_EDGE ( 'NONE', *, *, #6535, .T. ) ;
#1263=LINE ( 'NONE', #14523, #2893 ) ;
#1264=CARTESIAN_POINT ( 'NONE',  ( -76.50000000000001421, -179.3058001507315566, -51.45141194869120227 ) ) ;
#1265=AXIS2_PLACEMENT_3D ( 'NONE', #8938, #301, #14754 ) ;
#1267=EDGE_CURVE ( 'NONE', #3320, #3389, #13855, .T. ) ;
#1268=CARTESIAN_POINT ( 'NONE',  ( 190.0000000000000853, 16.03993994372673626, 52.49999999999997868 ) ) ;
#1271=CARTESIAN_POINT ( 'NONE',  ( 190.0000000000000568, 15.03993994372673981, -2.575184203610571654 ) ) ;
#1278=ORIENTED_EDGE ( 'NONE', *, *, #6461, .T. ) ;
#1279=ORIENTED_EDGE ( 'NONE', *, *, #10935, .F. ) ;
#1283=ORIENTED_EDGE ( 'NONE', *, *, #4940, .F. ) ;
#1284=DIRECTION ( 'NONE',  ( -2.897122145519000304E-15, -0.9902680687415702510, -0.1391731009600660485 ) ) ;
#1289=ORIENTED_EDGE ( 'NONE', *, *, #2581, .F. ) ;
#1293=DIRECTION ( 'NONE',  ( -1.000000000000000000, 0.000000000000000000, 0.000000000000000000 ) ) ;
#1297=ORIENTED_EDGE ( 'NONE', *, *, #3867, .T. ) ;
#1301=ORIENTED_EDGE ( 'NONE', *, *, #4197, .T. ) ;
#1304=DIRECTION ( 'NONE',  ( 0.000000000000000000, 1.000000000000000000, 0.000000000000000000 ) ) ;
#1310=EDGE_CURVE ( 'NONE', #2929, #12060, #10398, .T. ) ;
#1314=AXIS2_PLACEMENT_3D ( 'NONE', #11044, #9473, #2518 ) ;
#1323=CARTESIAN_POINT ( 'NONE',  ( -63.50000000000002842, 15.03993994372673981, 10.05257423913146475 ) ) ;
#1329=AXIS2_PLACEMENT_3D ( 'NONE', #12163, #3878, #2537 ) ;
#1330=ORIENTED_EDGE ( 'NONE', *, *, #8852, .T. ) ;
#1334=CIRCLE ( 'NONE', #10421, 0.5000000000000001110 ) ;
#1344=ADVANCED_FACE ( 'NONE', ( #14014 ), #5891, .T. ) ;
#1346=ORIENTED_EDGE ( 'NONE', *, *, #14428, .T. ) ;
#1347=AXIS2_PLACEMENT_3D ( 'NONE', #14029, #8142, #8292 ) ;
#1348=ORIENTED_EDGE ( 'NONE', *, *, #804, .T. ) ;
#1350=CARTESIAN_POINT ( 'NONE',  ( -64.00000000000002842, -178.8058001507315566, 52.19066787724494816 ) ) ;
#1353=ORIENTED_EDGE ( 'NONE', *, *, #12446, .F. ) ;
#1357=AXIS2_PLACEMENT_3D ( 'NONE', #383, #763, #10414 ) ;
#1358=VERTEX_POINT ( 'NONE', #7088 ) ;
#1360=CARTESIAN_POINT ( 'NONE',  ( 178.0000000000000853, -179.3058001507315566, -51.45141194869120227 ) ) ;
#1362=DIRECTION ( 'NONE',  ( 0.000000000000000000, 0.000000000000000000, -1.000000000000000000 ) ) ;
#1365=AXIS2_PLACEMENT_3D ( 'NONE', #660, #14086, #4220 ) ;
#1375=EDGE_LOOP ( 'NONE', ( #15098, #949, #3175, #1346 ) ) ;
#1376=ORIENTED_EDGE ( 'NONE', *, *, #7639, .F. ) ;
#1380=DIRECTION ( 'NONE',  ( 1.000000000000000000, -2.751328491981765035E-32, 3.965082230804130220E-16 ) ) ;
#1382=DIRECTION ( 'NONE',  ( 0.000000000000000000, -0.000000000000000000, 1.000000000000000000 ) ) ;
#1384=AXIS2_PLACEMENT_3D ( 'NONE', #4184, #7925, #11302 ) ;
#1390=EDGE_CURVE ( 'NONE', #14442, #4447, #3528, .T. ) ;
#1399=ADVANCED_FACE ( 'NONE', ( #14319 ), #2015, .F. ) ;
#1412=CIRCLE ( 'NONE', #10253, 0.5000000000000000000 ) ;
#1414=AXIS2_PLACEMENT_3D ( 'NONE', #7818, #12607, #6634 ) ;
#1416=ORIENTED_EDGE ( 'NONE', *, *, #11845, .F. ) ;
#1417=ADVANCED_FACE ( 'NONE', ( #13136 ), #14354, .T. ) ;
#1419=CARTESIAN_POINT ( 'NONE',  ( -76.00000000000004263, 16.03993994372673626, 52.49999999999997868 ) ) ;
#1431=ORIENTED_EDGE ( 'NONE', *, *, #9842, .T. ) ;
#1436=LINE ( 'NONE', #14853, #10494 ) ;
#1437=FACE_OUTER_BOUND ( 'NONE', #8455, .T. ) ;
#1438=AXIS2_PLACEMENT_3D ( 'NONE', #15216, #5529, #12694 ) ;
#1441=CARTESIAN_POINT ( 'NONE',  ( 190.5000000000000853, 15.53993994372673626, 52.49999999999997868 ) ) ;
#1450=ORIENTED_EDGE ( 'NONE', *, *, #14813, .F. ) ;
#1456=VECTOR ( 'NONE', #9861, 1000.000000000000000 ) ;
#1458=DIRECTION ( 'NONE',  ( 0.000000000000000000, 0.000000000000000000, 1.000000000000000000 ) ) ;
#1465=PLANE ( 'NONE',  #11873 ) ;
#1471=CARTESIAN_POINT ( 'NONE',  ( 184.0000000000000568, 17.53993994372673981, -12.49999999999999289 ) ) ;
#1474=DIRECTION ( 'NONE',  ( 0.000000000000000000, 0.000000000000000000, 1.000000000000000000 ) ) ;
#1475=DIRECTION ( 'NONE',  ( 0.000000000000000000, 0.000000000000000000, -1.000000000000000000 ) ) ;
#1479=EDGE_CURVE ( 'NONE', #9446, #12308, #13088, .T. ) ;
#1481=AXIS2_PLACEMENT_3D ( 'NONE', #13040, #2164, #11802 ) ;
#1482=VECTOR ( 'NONE', #15073, 1000.000000000000000 ) ;
#1483=DIRECTION ( 'NONE',  ( 1.000000000000000000, 0.000000000000000000, 0.000000000000000000 ) ) ;
#1487=ORIENTED_EDGE ( 'NONE', *, *, #13530, .T. ) ;
#1488=CIRCLE ( 'NONE', #11593, 0.4999999999999996114 ) ;
#1489=EDGE_CURVE ( 'NONE', #13203, #2702, #11899, .T. ) ;
#1491=ORIENTED_EDGE ( 'NONE', *, *, #8346, .T. ) ;
#1498=FACE_OUTER_BOUND ( 'NONE', #14969, .T. ) ;
#1501=AXIS2_PLACEMENT_3D ( 'NONE', #3784, #2757, #6235 ) ;
#1503=TOROIDAL_SURFACE ( 'NONE', #5559, 1.000000000000000000, 0.5000000000000000000 ) ;
#1504=ORIENTED_EDGE ( 'NONE', *, *, #3354, .F. ) ;
#1506=ADVANCED_FACE ( 'NONE', ( #11979 ), #5977, .F. ) ;
#1513=CIRCLE ( 'NONE', #7334, 0.5000000000000001110 ) ;
#1515=ORIENTED_EDGE ( 'NONE', *, *, #10550, .F. ) ;
#1518=AXIS2_PLACEMENT_3D ( 'NONE', #7907, #11599, #764 ) ;
#1520=DIRECTION ( 'NONE',  ( 0.000000000000000000, -3.469446951953611033E-15, 1.000000000000000000 ) ) ;
#1522=DIRECTION ( 'NONE',  ( 0.000000000000000000, 0.000000000000000000, 1.000000000000000000 ) ) ;
#1539=DIRECTION ( 'NONE',  ( 0.000000000000000000, 0.1391731009600584990, -0.9902680687415712502 ) ) ;
#1542=EDGE_CURVE ( 'NONE', #10751, #7203, #3606, .T. ) ;
#1543=AXIS2_PLACEMENT_3D ( 'NONE', #2647, #7468, #13284 ) ;
#1547=TOROIDAL_SURFACE ( 'NONE', #5330, 1.000000000000000000, 0.5000000000000000000 ) ;
#1550=LINE ( 'NONE', #3854, #9543 ) ;
#1555=ORIENTED_EDGE ( 'NONE', *, *, #1929, .F. ) ;
#1558=DIRECTION ( 'NONE',  ( 0.000000000000000000, 0.000000000000000000, -1.000000000000000000 ) ) ;
#1561=CARTESIAN_POINT ( 'NONE',  ( 190.5000000000000568, 16.03993994372673981, -17.50000000000002487 ) ) ;
#1562=CIRCLE ( 'NONE', #9643, 0.5000000000000004441 ) ;
#1567=EDGE_CURVE ( 'NONE', #6280, #14008, #35, .T. ) ;
#1568=DIRECTION ( 'NONE',  ( 0.000000000000000000, -1.000000000000000000, 0.000000000000000000 ) ) ;
#1572=VERTEX_POINT ( 'NONE', #8212 ) ;
#1576=ORIENTED_EDGE ( 'NONE', *, *, #11922, .F. ) ;
#1577=DIRECTION ( 'NONE',  ( 0.000000000000000000, -6.938893903907227145E-17, 1.000000000000000000 ) ) ;
#1578=CYLINDRICAL_SURFACE ( 'NONE', #3049, 1.499999999999997780 ) ;
#1581=ORIENTED_EDGE ( 'NONE', *, *, #8363, .T. ) ;
#1583=CIRCLE ( 'NONE', #7152, 0.5000000000000001110 ) ;
#1590=CIRCLE ( 'NONE', #10426, 0.5000000000000004441 ) ;
#1591=PLANE ( 'NONE',  #202 ) ;
#1592=VERTEX_POINT ( 'NONE', #8588 ) ;
#1596=ORIENTED_EDGE ( 'NONE', *, *, #13880, .T. ) ;
#1597=CARTESIAN_POINT ( 'NONE',  ( 178.0000000000000853, 15.03993994372673981, -2.575184203610571654 ) ) ;
#1600=DIRECTION ( 'NONE',  ( -0.000000000000000000, -0.000000000000000000, -1.000000000000000000 ) ) ;
#1602=EDGE_CURVE ( 'NONE', #15306, #9812, #3267, .T. ) ;
#1605=CARTESIAN_POINT ( 'NONE',  ( 190.0000000000000853, -179.8058001507315566, 84.88378295107887084 ) ) ;
#1606=AXIS2_PLACEMENT_3D ( 'NONE', #5249, #1539, #1695 ) ;
#1611=LINE ( 'NONE', #14705, #12641 ) ;
#1615=DIRECTION ( 'NONE',  ( -1.000000000000000000, 0.000000000000000000, 0.000000000000000000 ) ) ;
#1619=( GEOMETRIC_REPRESENTATION_CONTEXT ( 3 ) GLOBAL_UNCERTAINTY_ASSIGNED_CONTEXT ( ( #726 ) ) GLOBAL_UNIT_ASSIGNED_CONTEXT ( ( #3698, #15606, #6159 ) ) REPRESENTATION_CONTEXT ( 'NONE', 'WORKASPACE' ) );
#1626=LINE ( 'NONE', #11114, #3622 ) ;
#1631=VERTEX_POINT ( 'NONE', #5314 ) ;
#1632=DIRECTION ( 'NONE',  ( -1.000000000000000000, 0.000000000000000000, 0.000000000000000000 ) ) ;
#1637=CARTESIAN_POINT ( 'NONE',  ( -76.50000000000004263, 15.60952649420676686, 25.87720316414728217 ) ) ;
#1642=DIRECTION ( 'NONE',  ( -0.000000000000000000, -4.956352788505162775E-17, 1.000000000000000000 ) ) ;
#1657=CARTESIAN_POINT ( 'NONE',  ( -76.00000000000004263, 15.03993994372673804, 38.07518420361041933 ) ) ;
#1658=LINE ( 'NONE', #14827, #7342 ) ;
#1661=ORIENTED_EDGE ( 'NONE', *, *, #3705, .F. ) ;
#1663=ORIENTED_EDGE ( 'NONE', *, *, #1542, .T. ) ;
#1667=TOROIDAL_SURFACE ( 'NONE', #3685, 1.000000000000000000, 0.5000000000000000000 ) ;
#1669=AXIS2_PLACEMENT_3D ( 'NONE', #12201, #13386, #11188 ) ;
#1671=DIRECTION ( 'NONE',  ( 3.965082230804130220E-16, 0.000000000000000000, 1.000000000000000000 ) ) ;
#1677=DIRECTION ( 'NONE',  ( -3.965082230804130220E-16, 1.090924371466202084E-47, 1.000000000000000000 ) ) ;
#1679=DIRECTION ( 'NONE',  ( -0.000000000000000000, 0.9902680687415705840, 0.1391731009600641333 ) ) ;
#1680=CYLINDRICAL_SURFACE ( 'NONE', #15266, 1.500000000000001332 ) ;
#1693=ORIENTED_EDGE ( 'NONE', *, *, #657, .F. ) ;
#1695=DIRECTION ( 'NONE',  ( 0.000000000000000000, 0.9902680687415712502, 0.1391731009600584990 ) ) ;
#1696=DIRECTION ( 'NONE',  ( 0.000000000000000000, 4.956352788505162775E-17, -1.000000000000000000 ) ) ;
#1702=EDGE_CURVE ( 'NONE', #14752, #11943, #3760, .T. ) ;
#1704=CARTESIAN_POINT ( 'NONE',  ( -76.50000000000004263, 17.53993994372673626, 52.49999999999997868 ) ) ;
#1705=DIRECTION ( 'NONE',  ( 0.000000000000000000, 0.000000000000000000, -1.000000000000000000 ) ) ;
#1707=ORIENTED_EDGE ( 'NONE', *, *, #4864, .T. ) ;
#1709=ORIENTED_EDGE ( 'NONE', *, *, #11072, .F. ) ;
#1711=DIRECTION ( 'NONE',  ( -3.965082230804130220E-16, -4.956352788505162775E-17, 1.000000000000000000 ) ) ;
#1715=DIRECTION ( 'NONE',  ( 0.000000000000000000, 4.956352788505162775E-17, -1.000000000000000000 ) ) ;
#1720=TOROIDAL_SURFACE ( 'NONE', #10807, 1.000000000000000000, 0.5000000000000000000 ) ;
#1723=VECTOR ( 'NONE', #12040, 1000.000000000000000 ) ;
#1724=DIRECTION ( 'NONE',  ( 1.000000000000000000, -2.751328491981765035E-32, 3.965082230804130220E-16 ) ) ;
#1728=ORIENTED_EDGE ( 'NONE', *, *, #5273, .F. ) ;
#1730=CARTESIAN_POINT ( 'NONE',  ( 190.0000000000000568, -178.8058001507315566, 52.19066787724494816 ) ) ;
#1737=LINE ( 'NONE', #10040, #3352 ) ;
#1746=DIRECTION ( 'NONE',  ( 1.000000000000000000, -2.751328491981765035E-32, 3.965082230804130220E-16 ) ) ;
#1749=CARTESIAN_POINT ( 'NONE',  ( 177.5000000000000853, 17.53993994372673626, 52.49999999999997868 ) ) ;
#1758=CARTESIAN_POINT ( 'NONE',  ( 175.9483885134608272, 15.03993994372673804, 24.94742576086838781 ) ) ;
#1762=CIRCLE ( 'NONE', #10603, 0.5000000000000004441 ) ;
#1763=EDGE_LOOP ( 'NONE', ( #6689, #9777, #2063, #3637, #11582, #11850 ) ) ;
#1764=EDGE_CURVE ( 'NONE', #10201, #15193, #1762, .T. ) ;
#1766=CIRCLE ( 'NONE', #10604, 0.4999999999999996114 ) ;
#1769=ORIENTED_EDGE ( 'NONE', *, *, #4176, .F. ) ;
#1772=EDGE_LOOP ( 'NONE', ( #14110, #1416, #2018, #11573, #13939 ) ) ;
#1774=DIRECTION ( 'NONE',  ( 0.000000000000000000, 0.000000000000000000, 1.000000000000000000 ) ) ;
#1775=CIRCLE ( 'NONE', #12365, 0.5000000000000000000 ) ;
#1786=AXIS2_PLACEMENT_3D ( 'NONE', #554, #15078, #1828 ) ;
#1789=ORIENTED_EDGE ( 'NONE', *, *, #14718, .T. ) ;
#1790=DIRECTION ( 'NONE',  ( -3.965082230804130220E-16, 0.000000000000000000, -1.000000000000000000 ) ) ;
#1791=DIRECTION ( 'NONE',  ( 0.000000000000000000, 0.000000000000000000, -1.000000000000000000 ) ) ;
#1795=EDGE_CURVE ( 'NONE', #8082, #15155, #1002, .T. ) ;
#1797=EDGE_CURVE ( 'NONE', #14752, #6214, #9094, .T. ) ;
#1798=CARTESIAN_POINT ( 'NONE',  ( 177.5000000000000853, 15.03993994372673804, 38.07518420361041933 ) ) ;
#1807=VERTEX_POINT ( 'NONE', #12795 ) ;
#1808=DIRECTION ( 'NONE',  ( -1.000000000000000000, -2.751328491981765035E-32, 3.965082230804130220E-16 ) ) ;
#1813=CARTESIAN_POINT ( 'NONE',  ( 177.5000000000000853, -179.8058001507315566, -51.45141194869119516 ) ) ;
#1814=EDGE_LOOP ( 'NONE', ( #8734, #6895, #10209, #9391 ) ) ;
#1819=CARTESIAN_POINT ( 'NONE',  ( 178.0000000000000853, 15.03993994372673981, -3.075184203610571654 ) ) ;
#1823=DIRECTION ( 'NONE',  ( -5.518327896226364679E-17, 0.9902680687415713612, -0.1391731009600582492 ) ) ;
#1826=ORIENTED_EDGE ( 'NONE', *, *, #4772, .T. ) ;
#1828=DIRECTION ( 'NONE',  ( 0.000000000000000000, 0.000000000000000000, 1.000000000000000000 ) ) ;
#1830=EDGE_LOOP ( 'NONE', ( #15345, #10863, #12246, #390 ) ) ;
#1838=VERTEX_POINT ( 'NONE', #9266 ) ;
#1841=CARTESIAN_POINT ( 'NONE',  ( 178.0000000000000853, 15.53993994372673981, 25.38206912977650376 ) ) ;
#1845=VECTOR ( 'NONE', #11518, 1000.000000000000000 ) ;
#1846=EDGE_LOOP ( 'NONE', ( #10498, #6434, #10055, #11627, #4626, #13978 ) ) ;
#1852=AXIS2_PLACEMENT_3D ( 'NONE', #4069, #8904, #3849 ) ;
#1853=CARTESIAN_POINT ( 'NONE',  ( -76.00000000000004263, 15.03993994372673804, 38.07518420361041933 ) ) ;
#1854=ORIENTED_EDGE ( 'NONE', *, *, #11944, .T. ) ;
#1855=DIRECTION ( 'NONE',  ( 0.000000000000000000, 0.000000000000000000, -1.000000000000000000 ) ) ;
#1857=CARTESIAN_POINT ( 'NONE',  ( 190.0000000000000853, 16.03993994372673626, 38.07518420361041933 ) ) ;
#1858=DIRECTION ( 'NONE',  ( 1.000000000000000000, 0.000000000000000000, 0.000000000000000000 ) ) ;
#1860=LINE ( 'NONE', #2178, #9876 ) ;
#1864=LINE ( 'NONE', #15347, #13706 ) ;
#1865=DIRECTION ( 'NONE',  ( 0.000000000000000000, -6.938893903907222067E-15, 1.000000000000000000 ) ) ;
#1866=VECTOR ( 'NONE', #14338, 1000.000000000000000 ) ;
#1870=CARTESIAN_POINT ( 'NONE',  ( -70.00000000000000000, 17.53993994372673981, -13.99999999999999112 ) ) ;
#1871=CARTESIAN_POINT ( 'NONE',  ( -76.00000000000001421, -178.8058001507315566, 52.19066787724494816 ) ) ;
#1874=EDGE_CURVE ( 'NONE', #10895, #14008, #4279, .T. ) ;
#1875=DIRECTION ( 'NONE',  ( 1.000000000000000000, 0.000000000000000000, 0.000000000000000000 ) ) ;
#1885=CARTESIAN_POINT ( 'NONE',  ( -76.00000000000001421, 16.03993994372673981, -7.458121719691109004E-14 ) ) ;
#1893=CARTESIAN_POINT ( 'NONE',  ( 0.000000000000000000, 15.53993994372673981, 7.305634244248866343E-16 ) ) ;
#1897=EDGE_CURVE ( 'NONE', #7467, #12599, #1513, .T. ) ;
#1904=DIRECTION ( 'NONE',  ( 0.000000000000000000, 1.000000000000000000, 6.938893903907227145E-17 ) ) ;
#1913=VECTOR ( 'NONE', #13223, 1000.000000000000000 ) ;
#1914=CARTESIAN_POINT ( 'NONE',  ( 177.5000000000000853, 14.90076684276667862, -2.084916134868993076 ) ) ;
#1915=EDGE_LOOP ( 'NONE', ( #530, #360, #10507, #9850, #14863, #4420 ) ) ;
#1922=ORIENTED_EDGE ( 'NONE', *, *, #4578, .F. ) ;
#1926=EDGE_CURVE ( 'NONE', #830, #3704, #9593, .T. ) ;
#1929=EDGE_CURVE ( 'NONE', #10201, #12658, #2383, .T. ) ;
#1931=DIRECTION ( 'NONE',  ( 0.000000000000000000, 2.775557561562888827E-14, 1.000000000000000000 ) ) ;
#1934=LINE ( 'NONE', #11506, #11849 ) ;
#1935=ORIENTED_EDGE ( 'NONE', *, *, #8976, .T. ) ;
#1936=DIRECTION ( 'NONE',  ( 1.000000000000000000, -2.751328491981765035E-32, 3.965082230804130220E-16 ) ) ;
#1944=CARTESIAN_POINT ( 'NONE',  ( 190.0000000000000568, -178.7362136002515172, -17.68580191161595394 ) ) ;
#1945=LINE ( 'NONE', #5518, #1845 ) ;
#1948=CARTESIAN_POINT ( 'NONE',  ( -61.94838851346079167, -179.3058001507315566, -51.45141194869120227 ) ) ;
#1950=CARTESIAN_POINT ( 'NONE',  ( 177.5000000000000853, -179.8058001507315566, 84.88378295107887084 ) ) ;
#1954=( NAMED_UNIT ( * ) SI_UNIT ( $, .STERADIAN. ) SOLID_ANGLE_UNIT ( ) );
#1955=VERTEX_POINT ( 'NONE', #12015 ) ;
#1956=CARTESIAN_POINT ( 'NONE',  ( 178.0000000000000853, -178.8058001507315566, -17.19066787724516843 ) ) ;
#1958=ORIENTED_EDGE ( 'NONE', *, *, #11334, .T. ) ;
#1963=AXIS2_PLACEMENT_3D ( 'NONE', #9341, #14136, #11472 ) ;
#1964=DIRECTION ( 'NONE',  ( 0.000000000000000000, 0.000000000000000000, 1.000000000000000000 ) ) ;
#1965=ORIENTED_EDGE ( 'NONE', *, *, #9339, .F. ) ;
#1967=EDGE_CURVE ( 'NONE', #5844, #1807, #3233, .T. ) ;
#1968=SHAPE_DEFINITION_REPRESENTATION ( #564, #8648 ) ;
#1969=ORIENTED_EDGE ( 'NONE', *, *, #12096, .T. ) ;
#1972=ORIENTED_EDGE ( 'NONE', *, *, #10428, .T. ) ;
#1973=CARTESIAN_POINT ( 'NONE',  ( 178.0000000000000853, 15.53993994372673981, 10.05257423913146475 ) ) ;
#1975=DIRECTION ( 'NONE',  ( 1.000000000000000000, 0.000000000000000000, 0.000000000000000000 ) ) ;
#1976=ORIENTED_EDGE ( 'NONE', *, *, #7499, .F. ) ;
#1983=DIRECTION ( 'NONE',  ( -0.000000000000000000, -0.000000000000000000, 1.000000000000000000 ) ) ;
#1984=DIRECTION ( 'NONE',  ( 0.000000000000000000, 0.000000000000000000, 1.000000000000000000 ) ) ;
#1986=DIRECTION ( 'NONE',  ( 1.000000000000000000, -2.751328491981765035E-32, 3.965082230804130220E-16 ) ) ;
#1989=EDGE_CURVE ( 'NONE', #2929, #13434, #7442, .T. ) ;
#1990=AXIS2_PLACEMENT_3D ( 'NONE', #15444, #3390, #13315 ) ;
#1996=DIRECTION ( 'NONE',  ( 0.000000000000000000, 0.1391731009600582492, 0.9902680687415713612 ) ) ;
#2003=EDGE_CURVE ( 'NONE', #8877, #652, #12086, .T. ) ;
#2005=FACE_OUTER_BOUND ( 'NONE', #9338, .T. ) ;
#2006=DIRECTION ( 'NONE',  ( 0.000000000000000000, -1.000000000000000000, 0.000000000000000000 ) ) ;
#2012=CARTESIAN_POINT ( 'NONE',  ( -63.50000000000002842, -178.8058001507315566, -17.19066787724516843 ) ) ;
#2015=CYLINDRICAL_SURFACE ( 'NONE', #11093, 0.5000000000000004441 ) ;
#2017=DIRECTION ( 'NONE',  ( -0.000000000000000000, 0.1391731009600582492, 0.9902680687415713612 ) ) ;
#2018=ORIENTED_EDGE ( 'NONE', *, *, #4319, .F. ) ;
#2019=ADVANCED_FACE ( 'NONE', ( #9731 ), #6016, .T. ) ;
#2020=ORIENTED_EDGE ( 'NONE', *, *, #1479, .F. ) ;
#2023=DIRECTION ( 'NONE',  ( 0.000000000000000000, -1.000000000000000000, 0.000000000000000000 ) ) ;
#2025=EDGE_CURVE ( 'NONE', #3026, #5369, #6087, .T. ) ;
#2027=DIRECTION ( 'NONE',  ( 0.000000000000000000, 0.1391731009600592484, 0.9902680687415712502 ) ) ;
#2028=CARTESIAN_POINT ( 'NONE',  ( 175.9483885134608272, -179.3058001507315566, -51.45141194869120227 ) ) ;
#2032=CIRCLE ( 'NONE', #3551, 0.5000000000000004441 ) ;
#2035=DIRECTION ( 'NONE',  ( 1.504267769033196424E-15, 0.9902680687415713612, 0.1391731009600591373 ) ) ;
#2040=FACE_OUTER_BOUND ( 'NONE', #13110, .T. ) ;
#2043=DIRECTION ( 'NONE',  ( 3.965082230804130220E-16, 1.090924371466202084E-47, 1.000000000000000000 ) ) ;
#2049=VERTEX_POINT ( 'NONE', #10994 ) ;
#2056=DIRECTION ( 'NONE',  ( 0.000000000000000000, 0.000000000000000000, -1.000000000000000000 ) ) ;
#2057=ORIENTED_EDGE ( 'NONE', *, *, #6303, .F. ) ;
#2060=CARTESIAN_POINT ( 'NONE',  ( -76.50000000000001421, -178.8058001507315566, -17.19066787724516843 ) ) ;
#2062=EDGE_CURVE ( 'NONE', #6505, #10500, #2539, .T. ) ;
#2063=ORIENTED_EDGE ( 'NONE', *, *, #7722, .F. ) ;
#2064=CYLINDRICAL_SURFACE ( 'NONE', #15551, 0.5000000000000004441 ) ;
#2065=CARTESIAN_POINT ( 'NONE',  ( -76.00000000000001421, 16.03993994372673981, 10.05257423913146475 ) ) ;
#2068=CARTESIAN_POINT ( 'NONE',  ( -70.00000000000000000, 17.53993994372673626, 47.49999999999997868 ) ) ;
#2071=CIRCLE ( 'NONE', #7884, 0.5000000000000004441 ) ;
#2072=VECTOR ( 'NONE', #11351, 1000.000000000000000 ) ;
#2078=ORIENTED_EDGE ( 'NONE', *, *, #15014, .T. ) ;
#2082=EDGE_CURVE ( 'NONE', #3561, #720, #11065, .T. ) ;
#2088=EDGE_CURVE ( 'NONE', #7203, #4389, #11625, .T. ) ;
#2091=ORIENTED_EDGE ( 'NONE', *, *, #3486, .F. ) ;
#2095=ORIENTED_EDGE ( 'NONE', *, *, #14233, .F. ) ;
#2097=VECTOR ( 'NONE', #15046, 1000.000000000000114 ) ;
#2105=FACE_OUTER_BOUND ( 'NONE', #610, .T. ) ;
#2111=ADVANCED_FACE ( 'NONE', ( #6334 ), #8858, .T. ) ;
#2116=ADVANCED_FACE ( 'NONE', ( #5293 ), #1578, .F. ) ;
#2123=STYLED_ITEM ( 'NONE', ( #4412 ), #5438 ) ;
#2128=AXIS2_PLACEMENT_3D ( 'NONE', #13133, #3596, #10946 ) ;
#2131=EDGE_CURVE ( 'NONE', #1137, #10552, #6843, .T. ) ;
#2135=CARTESIAN_POINT ( 'NONE',  ( 0.000000000000000000, 15.53993994372673981, 7.305634244248866343E-16 ) ) ;
#2143=DIRECTION ( 'NONE',  ( -1.000000000000000000, 0.000000000000000000, 0.000000000000000000 ) ) ;
#2144=CARTESIAN_POINT ( 'NONE',  ( 184.0000000000000568, 15.53993994372673626, 47.49999999999997868 ) ) ;
#2147=VECTOR ( 'NONE', #6810, 1000.000000000000000 ) ;
#2151=AXIS2_PLACEMENT_3D ( 'NONE', #14466, #9590, #14388 ) ;
#2152=LINE ( 'NONE', #1188, #13732 ) ;
#2153=CARTESIAN_POINT ( 'NONE',  ( -64.00000000000002842, 15.03993994372673981, -2.575184203610571654 ) ) ;
#2154=FACE_OUTER_BOUND ( 'NONE', #3928, .T. ) ;
#2162=TOROIDAL_SURFACE ( 'NONE', #3174, 1.000000000000000000, 0.5000000000000000000 ) ;
#2164=DIRECTION ( 'NONE',  ( 0.000000000000000000, 0.000000000000000000, -1.000000000000000000 ) ) ;
#2167=EDGE_CURVE ( 'NONE', #138, #12060, #13112, .T. ) ;
#2178=CARTESIAN_POINT ( 'NONE',  ( -76.50000000000001421, 17.53993994372673981, -17.50000000000002487 ) ) ;
#2179=CIRCLE ( 'NONE', #8249, 1.499999999999994449 ) ;
#2182=DIRECTION ( 'NONE',  ( 0.000000000000000000, 0.000000000000000000, -1.000000000000000000 ) ) ;
#2185=CARTESIAN_POINT ( 'NONE',  ( 175.9483885134608272, -179.3058001507315566, -17.76585208085566947 ) ) ;
#2188=EDGE_CURVE ( 'NONE', #8586, #1572, #1658, .T. ) ;
#2193=CARTESIAN_POINT ( 'NONE',  ( -64.00000000000002842, 14.90076684276668040, -2.084916134869000182 ) ) ;
#2194=CARTESIAN_POINT ( 'NONE',  ( -76.50000000000001421, 14.97035339324670922, -2.580050169239785696 ) ) ;
#2200=CARTESIAN_POINT ( 'NONE',  ( -64.00000000000002842, 15.03993994372673804, 38.07518420361041933 ) ) ;
#2202=LINE ( 'NONE', #5913, #10890 ) ;
#2209=TOROIDAL_SURFACE ( 'NONE', #683, 1.000000000000000000, 0.5000000000000000000 ) ;
#2213=EDGE_LOOP ( 'NONE', ( #2493, #9022, #3912, #7323, #9627 ) ) ;
#2214=DIRECTION ( 'NONE',  ( 0.000000000000000000, 0.000000000000000000, 1.000000000000000000 ) ) ;
#2220=VERTEX_POINT ( 'NONE', #13494 ) ;
#2221=AXIS2_PLACEMENT_3D ( 'NONE', #4392, #8047, #15272 ) ;
#2225=LINE ( 'NONE', #4987, #6382 ) ;
#2226=EDGE_LOOP ( 'NONE', ( #11645, #7359, #12227, #1854 ) ) ;
#2227=AXIS2_PLACEMENT_3D ( 'NONE', #510, #15040, #6392 ) ;
#2229=CARTESIAN_POINT ( 'NONE',  ( 178.0000000000000853, 15.53993994372673981, -2.500000000000070610 ) ) ;
#2233=DIRECTION ( 'NONE',  ( 0.000000000000000000, 0.000000000000000000, 1.000000000000000000 ) ) ;
#2239=CARTESIAN_POINT ( 'NONE',  ( -64.00000000000002842, -178.6666270497714777, -18.18093594598673945 ) ) ;
#2243=VECTOR ( 'NONE', #15562, 1000.000000000000000 ) ;
#2245=ORIENTED_EDGE ( 'NONE', *, *, #11257, .F. ) ;
#2246=EDGE_CURVE ( 'NONE', #8808, #9261, #8232, .T. ) ;
#2250=CARTESIAN_POINT ( 'NONE',  ( 190.5000000000000568, -179.8058001507315566, -29.88378295107906624 ) ) ;
#2253=LINE ( 'NONE', #15574, #2995 ) ;
#2258=ORIENTED_EDGE ( 'NONE', *, *, #8099, .F. ) ;
#2270=DIRECTION ( 'NONE',  ( 0.000000000000000000, 0.1391731009600660485, -0.9902680687415702510 ) ) ;
#2272=CYLINDRICAL_SURFACE ( 'NONE', #431, 0.4999999999999996114 ) ;
#2278=EDGE_LOOP ( 'NONE', ( #2374, #13185 ) ) ;
#2281=ADVANCED_FACE ( 'NONE', ( #7036 ), #14041, .T. ) ;
#2285=EDGE_CURVE ( 'NONE', #15155, #7716, #15220, .T. ) ;
#2290=ORIENTED_EDGE ( 'NONE', *, *, #3840, .T. ) ;
#2297=ORIENTED_EDGE ( 'NONE', *, *, #549, .F. ) ;
#2298=DIRECTION ( 'NONE',  ( 0.000000000000000000, -0.9902680687415713612, 0.1391731009600582492 ) ) ;
#2300=VECTOR ( 'NONE', #3480, 1000.000000000000000 ) ;
#2304=VECTOR ( 'NONE', #12784, 1000.000000000000000 ) ;
#2308=ORIENTED_EDGE ( 'NONE', *, *, #12304, .F. ) ;
#2309=DIRECTION ( 'NONE',  ( 1.000000000000000000, 0.000000000000000000, 0.000000000000000000 ) ) ;
#2310=AXIS2_PLACEMENT_3D ( 'NONE', #10496, #7027, #1003 ) ;
#2312=EDGE_LOOP ( 'NONE', ( #1237, #13218, #15094, #2290 ) ) ;
#2313=CARTESIAN_POINT ( 'NONE',  ( -70.00000000000000000, 15.53993994372673981, -12.49999999999999289 ) ) ;
#2314=EDGE_CURVE ( 'NONE', #2984, #13426, #3159, .T. ) ;
#2318=ORIENTED_EDGE ( 'NONE', *, *, #3155, .F. ) ;
#2327=CARTESIAN_POINT ( 'NONE',  ( 178.0000000000000853, 15.03993994372673804, 37.57518420361041933 ) ) ;
#2328=EDGE_LOOP ( 'NONE', ( #14742, #2416, #6007, #15228 ) ) ;
#2333=ORIENTED_EDGE ( 'NONE', *, *, #2062, .F. ) ;
#2343=ORIENTED_EDGE ( 'NONE', *, *, #13260, .T. ) ;
#2344=DIRECTION ( 'NONE',  ( 0.000000000000000000, 1.000000000000000000, 0.000000000000000000 ) ) ;
#2347=PLANE ( 'NONE',  #10254 ) ;
#2350=DIRECTION ( 'NONE',  ( 1.000000000000000000, -0.000000000000000000, -0.000000000000000000 ) ) ;
#2352=EDGE_CURVE ( 'NONE', #1955, #4389, #2032, .T. ) ;
#2355=VERTEX_POINT ( 'NONE', #10502 ) ;
#2357=CARTESIAN_POINT ( 'NONE',  ( -64.00000000000002842, 15.03993994372673804, 38.07518420361041933 ) ) ;
#2360=CARTESIAN_POINT ( 'NONE',  ( 184.0000000000000568, -181.3058001507315566, -42.95141194869119516 ) ) ;
#2363=DIRECTION ( 'NONE',  ( 0.000000000000000000, -6.938893903907222067E-15, 1.000000000000000000 ) ) ;
#2368=ORIENTED_EDGE ( 'NONE', *, *, #823, .T. ) ;
#2372=EDGE_CURVE ( 'NONE', #12019, #9039, #1775, .T. ) ;
#2374=ORIENTED_EDGE ( 'NONE', *, *, #6336, .F. ) ;
#2378=EDGE_CURVE ( 'NONE', #7650, #12538, #5577, .T. ) ;
#2379=ORIENTED_EDGE ( 'NONE', *, *, #9833, .F. ) ;
#2380=LINE ( 'NONE', #9727, #15592 ) ;
#2381=CARTESIAN_POINT ( 'NONE',  ( 190.5000000000000853, 16.03993994372673626, 37.49999999999991473 ) ) ;
#2383=LINE ( 'NONE', #3643, #7585 ) ;
#2384=VECTOR ( 'NONE', #5148, 1000.000000000000000 ) ;
#2390=CARTESIAN_POINT ( 'NONE',  ( 178.0000000000000853, -179.8058001507315566, -17.19066787724516843 ) ) ;
#2393=LINE ( 'NONE', #2631, #15595 ) ;
#2394=VERTEX_POINT ( 'NONE', #4574 ) ;
#2399=CARTESIAN_POINT ( 'NONE',  ( -76.00000000000001421, 15.03993994372673981, 10.05257423913146475 ) ) ;
#2403=VECTOR ( 'NONE', #11486, 1000.000000000000000 ) ;
#2407=VERTEX_POINT ( 'NONE', #11611 ) ;
#2409=DIRECTION ( 'NONE',  ( 1.000000000000000000, 0.000000000000000000, 0.000000000000000000 ) ) ;
#2416=ORIENTED_EDGE ( 'NONE', *, *, #714, .T. ) ;
#2417=APPLICATION_CONTEXT ( 'automotive_design' ) ;
#2420=DIRECTION ( 'NONE',  ( 1.000000000000000000, 2.751328491981765035E-32, -3.965082230804130220E-16 ) ) ;
#2422=CARTESIAN_POINT ( 'NONE',  ( 177.5000000000000853, 16.03993994372673981, -2.500000000000071498 ) ) ;
#2423=CARTESIAN_POINT ( 'NONE',  ( -61.94838851346079167, -179.3058001507315566, 52.76585208085545275 ) ) ;
#2429=CIRCLE ( 'NONE', #1414, 0.5000000000000004441 ) ;
#2431=FACE_OUTER_BOUND ( 'NONE', #10418, .T. ) ;
#2443=EDGE_CURVE ( 'NONE', #5220, #9609, #399, .T. ) ;
#2444=ORIENTED_EDGE ( 'NONE', *, *, #11456, .F. ) ;
#2446=EDGE_LOOP ( 'NONE', ( #15223, #11561, #11556, #13688 ) ) ;
#2454=VERTEX_POINT ( 'NONE', #6084 ) ;
#2458=DIRECTION ( 'NONE',  ( 1.000000000000000000, 0.000000000000000000, 0.000000000000000000 ) ) ;
#2459=ORIENTED_EDGE ( 'NONE', *, *, #12208, .T. ) ;
#2461=FACE_OUTER_BOUND ( 'NONE', #10931, .T. ) ;
#2463=DIRECTION ( 'NONE',  ( 0.000000000000000000, 0.9902680687415713612, -0.1391731009600582492 ) ) ;
#2464=CIRCLE ( 'NONE', #10537, 1.500000000000001332 ) ;
#2466=DIRECTION ( 'NONE',  ( 0.000000000000000000, 0.000000000000000000, 1.000000000000000000 ) ) ;
#2471=AXIS2_PLACEMENT_3D ( 'NONE', #1350, #8631, #13427 ) ;
#2479=VECTOR ( 'NONE', #14694, 1000.000000000000000 ) ;
#2480=VERTEX_POINT ( 'NONE', #7200 ) ;
#2493=ORIENTED_EDGE ( 'NONE', *, *, #12725, .T. ) ;
#2494=ORIENTED_EDGE ( 'NONE', *, *, #1795, .T. ) ;
#2504=DIRECTION ( 'NONE',  ( 0.000000000000000000, -0.9902680687415714722, 0.1391731009600582769 ) ) ;
#2510=EDGE_LOOP ( 'NONE', ( #14634, #5325, #7397, #7546 ) ) ;
#2513=EDGE_LOOP ( 'NONE', ( #6791, #745, #3131, #3579, #74, #985, #2095, #13502, #11369 ) ) ;
#2516=DIRECTION ( 'NONE',  ( 0.000000000000000000, -1.734723475976808672E-15, -1.000000000000000000 ) ) ;
#2518=DIRECTION ( 'NONE',  ( 3.965082230804130220E-16, 1.090924371466202084E-47, 1.000000000000000000 ) ) ;
#2530=CARTESIAN_POINT ( 'NONE',  ( 190.0000000000000568, -179.3058001507315566, -17.19066787724516843 ) ) ;
#2534=DIRECTION ( 'NONE',  ( 0.000000000000000000, 0.000000000000000000, 1.000000000000000000 ) ) ;
#2537=DIRECTION ( 'NONE',  ( 0.000000000000000000, -0.1391731009600591096, 0.9902680687415711391 ) ) ;
#2538=DIRECTION ( 'NONE',  ( -1.000000000000000000, 0.000000000000000000, 0.000000000000000000 ) ) ;
#2539=CIRCLE ( 'NONE', #5064, 0.5000000000000004441 ) ;
#2540=EDGE_CURVE ( 'NONE', #15212, #5473, #4448, .T. ) ;
#2546=ORIENTED_EDGE ( 'NONE', *, *, #12587, .F. ) ;
#2549=CARTESIAN_POINT ( 'NONE',  ( 190.5000000000000853, 14.90076684276667507, 37.08491613486882699 ) ) ;
#2571=DIRECTION ( 'NONE',  ( 0.000000000000000000, 1.000000000000000000, 6.938893903907227145E-17 ) ) ;
#2572=EDGE_CURVE ( 'NONE', #2702, #6505, #12293, .T. ) ;
#2575=ORIENTED_EDGE ( 'NONE', *, *, #2352, .T. ) ;
#2577=AXIS2_PLACEMENT_3D ( 'NONE', #13721, #5363, #13638 ) ;
#2580=EDGE_LOOP ( 'NONE', ( #5296, #14213, #11579, #14953 ) ) ;
#2581=EDGE_CURVE ( 'NONE', #6993, #3478, #919, .T. ) ;
#2582=AXIS2_PLACEMENT_3D ( 'NONE', #10909, #3708, #8537 ) ;
#2584=DIRECTION ( 'NONE',  ( 0.000000000000000000, 0.000000000000000000, -1.000000000000000000 ) ) ;
#2585=CARTESIAN_POINT ( 'NONE',  ( -70.00000000000000000, 15.53993994372673626, 48.99999999999997158 ) ) ;
#2594=ORIENTED_EDGE ( 'NONE', *, *, #3965, .T. ) ;
#2600=DIRECTION ( 'NONE',  ( 0.000000000000000000, 0.000000000000000000, -1.000000000000000000 ) ) ;
#2603=DIRECTION ( 'NONE',  ( -1.000000000000000000, 0.000000000000000000, 0.000000000000000000 ) ) ;
#2606=EDGE_CURVE ( 'NONE', #7302, #13797, #1412, .T. ) ;
#2628=CARTESIAN_POINT ( 'NONE',  ( -76.50000000000001421, -178.9449732516916072, -29.32815825124561471 ) ) ;
#2631=CARTESIAN_POINT ( 'NONE',  ( 190.5000000000000568, 15.10952649420676686, 25.44255979523916977 ) ) ;
#2632=ORIENTED_EDGE ( 'NONE', *, *, #8001, .T. ) ;
#2633=ORIENTED_EDGE ( 'NONE', *, *, #15205, .F. ) ;
#2641=ADVANCED_FACE ( 'NONE', ( #5123, #10175 ), #7740, .T. ) ;
#2643=AXIS2_PLACEMENT_3D ( 'NONE', #9058, #10474, #5423 ) ;
#2647=CARTESIAN_POINT ( 'NONE',  ( -64.00000000000002842, -179.8058001507315566, -17.19066787724516843 ) ) ;
#2651=ORIENTED_EDGE ( 'NONE', *, *, #4189, .T. ) ;
#2656=EDGE_CURVE ( 'NONE', #1137, #235, #6474, .T. ) ;
#2657=VECTOR ( 'NONE', #5887, 1000.000000000000000 ) ;
#2660=CARTESIAN_POINT ( 'NONE',  ( 190.5000000000000853, 15.53993994372673626, 52.49999999999997868 ) ) ;
#2663=EDGE_CURVE ( 'NONE', #2049, #7175, #10775, .T. ) ;
#2668=DIRECTION ( 'NONE',  ( 1.000000000000000000, -2.751328491981765035E-32, 3.965082230804130220E-16 ) ) ;
#2672=CYLINDRICAL_SURFACE ( 'NONE', #9111, 0.5000000000000004441 ) ;
#2677=CARTESIAN_POINT ( 'NONE',  ( 190.5000000000000568, 15.53993994372673804, 38.07518420361041933 ) ) ;
#2679=CARTESIAN_POINT ( 'NONE',  ( -76.00000000000007105, -179.3058001507315566, 84.88378295107887084 ) ) ;
#2682=EDGE_CURVE ( 'NONE', #11943, #3320, #515, .T. ) ;
#2686=DIRECTION ( 'NONE',  ( 1.000000000000000000, -2.751328491981765035E-32, 3.965082230804130220E-16 ) ) ;
#2687=CARTESIAN_POINT ( 'NONE',  ( -76.50000000000004263, -178.8058001507315566, 65.31842631998698323 ) ) ;
#2689=VERTEX_POINT ( 'NONE', #7427 ) ;
#2691=ORIENTED_EDGE ( 'NONE', *, *, #11732, .F. ) ;
#2696=ORIENTED_EDGE ( 'NONE', *, *, #12610, .T. ) ;
#2699=FACE_BOUND ( 'NONE', #6003, .T. ) ;
#2700=ORIENTED_EDGE ( 'NONE', *, *, #12306, .T. ) ;
#2702=VERTEX_POINT ( 'NONE', #5045 ) ;
#2707=ADVANCED_FACE ( 'NONE', ( #9304 ), #14024, .T. ) ;
#2709=ORIENTED_EDGE ( 'NONE', *, *, #3577, .F. ) ;
#2710=EDGE_LOOP ( 'NONE', ( #11694, #3134, #10364, #520 ) ) ;
#2717=CIRCLE ( 'NONE', #9538, 1.499999999999997780 ) ;
#2722=CARTESIAN_POINT ( 'NONE',  ( -64.00000000000002842, -178.7362136002515172, -17.68580191161595394 ) ) ;
#2731=EDGE_LOOP ( 'NONE', ( #5610, #5692, #13217, #779 ) ) ;
#2736=EDGE_CURVE ( 'NONE', #11943, #13605, #2429, .T. ) ;
#2739=CARTESIAN_POINT ( 'NONE',  ( 190.0000000000000568, -179.3058001507315566, -30.31842631998718574 ) ) ;
#2741=VECTOR ( 'NONE', #13587, 1000.000000000000000 ) ;
#2743=CARTESIAN_POINT ( 'NONE',  ( -64.00000000000002842, -179.3058001507315566, -17.76585208085566947 ) ) ;
#2744=CYLINDRICAL_SURFACE ( 'NONE', #15165, 1.499999999999997780 ) ;
#2745=PRODUCT_DEFINITION_FORMATION_WITH_SPECIFIED_SOURCE ( 'ANY', '', #827, .NOT_KNOWN. ) ;
#2747=DIRECTION ( 'NONE',  ( 0.000000000000000000, -1.000000000000000000, -6.938893903907227145E-17 ) ) ;
#2748=AXIS2_PLACEMENT_3D ( 'NONE', #12654, #6685, #5324 ) ;
#2749=EDGE_CURVE ( 'NONE', #13177, #8794, #3687, .T. ) ;
#2754=LINE ( 'NONE', #13547, #6102 ) ;
#2756=DIRECTION ( 'NONE',  ( 0.000000000000000000, -1.000000000000000000, -4.956352788505162775E-17 ) ) ;
#2757=DIRECTION ( 'NONE',  ( 1.000000000000000000, -0.000000000000000000, -0.000000000000000000 ) ) ;
#2759=TOROIDAL_SURFACE ( 'NONE', #1438, 1.000000000000000000, 0.5000000000000000000 ) ;
#2760=EDGE_LOOP ( 'NONE', ( #481, #636, #11539, #11295 ) ) ;
#2762=CARTESIAN_POINT ( 'NONE',  ( -76.50000000000004263, 16.03993994372673626, 52.49999999999997868 ) ) ;
#2766=EDGE_CURVE ( 'NONE', #1572, #4643, #12131, .T. ) ;
#2767=AXIS2_PLACEMENT_3D ( 'NONE', #14539, #14465, #5005 ) ;
#2775=ORIENTED_EDGE ( 'NONE', *, *, #1077, .F. ) ;
#2777=CARTESIAN_POINT ( 'NONE',  ( 184.0000000000000568, 15.53993994372673981, -12.49999999999999289 ) ) ;
#2778=AXIS2_PLACEMENT_3D ( 'NONE', #15501, #4698, #4460 ) ;
#2779=CYLINDRICAL_SURFACE ( 'NONE', #9655, 1.499999999999994449 ) ;
#2786=ORIENTED_EDGE ( 'NONE', *, *, #6303, .T. ) ;
#2791=EDGE_LOOP ( 'NONE', ( #13497, #12888, #1976, #8409, #9800, #11347, #11896, #12895, #10326, #8554, #14802, #14242, #5073, #13272, #96, #7229, #10930 ) ) ;
#2795=ORIENTED_EDGE ( 'NONE', *, *, #10101, .F. ) ;
#2796=TOROIDAL_SURFACE ( 'NONE', #5053, 1.000000000000000000, 0.5000000000000000000 ) ;
#2798=EDGE_CURVE ( 'NONE', #85, #7982, #2179, .T. ) ;
#2799=DIRECTION ( 'NONE',  ( -0.000000000000000000, -1.000000000000000000, -0.000000000000000000 ) ) ;
#2807=FACE_OUTER_BOUND ( 'NONE', #9112, .T. ) ;
#2810=CARTESIAN_POINT ( 'NONE',  ( -64.00000000000002842, 16.03993994372673981, 24.94742576086838781 ) ) ;
#2816=DIRECTION ( 'NONE',  ( -0.000000000000000000, -0.000000000000000000, 1.000000000000000000 ) ) ;
#2819=CARTESIAN_POINT ( 'NONE',  ( 190.0000000000000568, 15.03993994372673981, -3.075184203610571654 ) ) ;
#2820=ADVANCED_FACE ( 'NONE', ( #14486 ), #2347, .T. ) ;
#2822=EDGE_LOOP ( 'NONE', ( #3197, #10041, #9471, #12428 ) ) ;
#2827=VECTOR ( 'NONE', #14128, 1000.000000000000000 ) ;
#2842=ADVANCED_FACE ( 'NONE', ( #7097 ), #9616, .T. ) ;
#2847=ORIENTED_EDGE ( 'NONE', *, *, #13348, .T. ) ;
#2855=DIRECTION ( 'NONE',  ( 0.000000000000000000, 0.000000000000000000, 1.000000000000000000 ) ) ;
#2858=ORIENTED_EDGE ( 'NONE', *, *, #12469, .T. ) ;
#2862=AXIS2_PLACEMENT_3D ( 'NONE', #14971, #2686, #6480 ) ;
#2864=ADVANCED_FACE ( 'NONE', ( #8443 ), #11902, .T. ) ;
#2866=VERTEX_POINT ( 'NONE', #3453 ) ;
#2872=DIRECTION ( 'NONE',  ( -1.000000000000000000, -0.000000000000000000, -0.000000000000000000 ) ) ;
#2876=DIRECTION ( 'NONE',  ( 5.518327896226369609E-17, -0.9902680687415712502, -0.1391731009600584990 ) ) ;
#2879=CARTESIAN_POINT ( 'NONE',  ( 184.0000000000000568, 17.53993994372673981, -13.99999999999999112 ) ) ;
#2889=DIRECTION ( 'NONE',  ( -0.000000000000000000, -0.000000000000000000, -1.000000000000000000 ) ) ;
#2893=VECTOR ( 'NONE', #6015, 1000.000000000000000 ) ;
#2896=FACE_OUTER_BOUND ( 'NONE', #5305, .T. ) ;
#2897=FACE_OUTER_BOUND ( 'NONE', #6854, .T. ) ;
#2899=AXIS2_PLACEMENT_3D ( 'NONE', #9214, #14011, #8036 ) ;
#2905=DIRECTION ( 'NONE',  ( 1.000000000000000000, 0.000000000000000000, 0.000000000000000000 ) ) ;
#2910=EDGE_LOOP ( 'NONE', ( #3757, #8169, #4486, #15269 ) ) ;
#2914=DIRECTION ( 'NONE',  ( -1.000000000000000000, 0.000000000000000000, 0.000000000000000000 ) ) ;
#2920=AXIS2_PLACEMENT_3D ( 'NONE', #8486, #15402, #4602 ) ;
#2926=ORIENTED_EDGE ( 'NONE', *, *, #9479, .T. ) ;
#2929=VERTEX_POINT ( 'NONE', #8284 ) ;
#2932=AXIS2_PLACEMENT_3D ( 'NONE', #8083, #5923, #14282 ) ;
#2934=CYLINDRICAL_SURFACE ( 'NONE', #5413, 0.5000000000000004441 ) ;
#2937=DIRECTION ( 'NONE',  ( 0.000000000000000000, -1.000000000000000000, 0.000000000000000000 ) ) ;
#2939=VERTEX_POINT ( 'NONE', #5181 ) ;
#2941=CARTESIAN_POINT ( 'NONE',  ( 190.0000000000000568, -178.8058001507315566, 52.19066787724494816 ) ) ;
#2943=DIRECTION ( 'NONE',  ( 0.000000000000000000, 0.000000000000000000, -1.000000000000000000 ) ) ;
#2945=LINE ( 'NONE', #10130, #1482 ) ;
#2952=CARTESIAN_POINT ( 'NONE',  ( -76.00000000000001421, -178.8058001507315566, 52.19066787724494816 ) ) ;
#2954=DIRECTION ( 'NONE',  ( 1.000000000000000000, -2.751328491981765035E-32, 3.965082230804130220E-16 ) ) ;
#2968=ADVANCED_FACE ( 'NONE', ( #12508, #12432, #8590 ), #3983, .F. ) ;
#2970=DIRECTION ( 'NONE',  ( 5.518327896226364679E-17, 0.9902680687415713612, -0.1391731009600582492 ) ) ;
#2971=DIRECTION ( 'NONE',  ( 0.000000000000000000, -4.956352788505162775E-17, 1.000000000000000000 ) ) ;
#2980=EDGE_LOOP ( 'NONE', ( #8266, #12008, #4748, #7928, #7781, #10017, #1254, #1301, #11027, #12713, #5802, #4416, #8024, #15559, #151, #9887, #4018 ) ) ;
#2982=AXIS2_PLACEMENT_3D ( 'NONE', #5268, #12522, #122 ) ;
#2983=ORIENTED_EDGE ( 'NONE', *, *, #14542, .T. ) ;
#2984=VERTEX_POINT ( 'NONE', #4065 ) ;
#2987=AXIS2_PLACEMENT_3D ( 'NONE', #6893, #5770, #10596 ) ;
#2991=DIRECTION ( 'NONE',  ( 1.000000000000000000, -0.000000000000000000, -0.000000000000000000 ) ) ;
#2992=AXIS2_PLACEMENT_3D ( 'NONE', #2068, #11921, #15610 ) ;
#2995=VECTOR ( 'NONE', #11739, 1000.000000000000000 ) ;
#3002=DIRECTION ( 'NONE',  ( 0.000000000000000000, 0.000000000000000000, -1.000000000000000000 ) ) ;
#3007=VECTOR ( 'NONE', #11348, 1000.000000000000114 ) ;
#3008=VECTOR ( 'NONE', #70, 1000.000000000000000 ) ;
#3009=AXIS2_PLACEMENT_3D ( 'NONE', #13350, #10767, #15553 ) ;
#3010=DIRECTION ( 'NONE',  ( 0.000000000000000000, 0.000000000000000000, -1.000000000000000000 ) ) ;
#3016=DIRECTION ( 'NONE',  ( 0.000000000000000000, 0.000000000000000000, 1.000000000000000000 ) ) ;
#3017=EDGE_LOOP ( 'NONE', ( #8521, #14268, #10102, #885 ) ) ;
#3018=FACE_OUTER_BOUND ( 'NONE', #708, .T. ) ;
#3020=LINE ( 'NONE', #465, #8570 ) ;
#3024=ADVANCED_FACE ( 'NONE', ( #3915 ), #341, .F. ) ;
#3025=DIRECTION ( 'NONE',  ( -0.000000000000000000, 0.9902680687415711391, -0.1391731009600603308 ) ) ;
#3026=VERTEX_POINT ( 'NONE', #2585 ) ;
#3029=AXIS2_PLACEMENT_3D ( 'NONE', #14409, #2420, #7253 ) ;
#3034=AXIS2_PLACEMENT_3D ( 'NONE', #477, #7623, #11089 ) ;
#3038=ORIENTED_EDGE ( 'NONE', *, *, #12446, .T. ) ;
#3039=CARTESIAN_POINT ( 'NONE',  ( 175.9483885134608272, -179.3058001507315566, 84.88378295107887084 ) ) ;
#3041=VECTOR ( 'NONE', #11189, 1000.000000000000000 ) ;
#3043=EDGE_LOOP ( 'NONE', ( #3329, #8841 ) ) ;
#3049=AXIS2_PLACEMENT_3D ( 'NONE', #2777, #9889, #7839 ) ;
#3056=DIRECTION ( 'NONE',  ( 0.000000000000000000, 0.000000000000000000, -1.000000000000000000 ) ) ;
#3066=AXIS2_PLACEMENT_3D ( 'NONE', #4001, #8835, #9601 ) ;
#3068=DIRECTION ( 'NONE',  ( -0.000000000000000000, -1.000000000000000000, -6.938893903907222067E-15 ) ) ;
#3072=CIRCLE ( 'NONE', #9374, 1.000000000000000888 ) ;
#3074=ADVANCED_FACE ( 'NONE', ( #2897 ), #4701, .T. ) ;
#3075=CARTESIAN_POINT ( 'NONE',  ( -70.00000000000000000, 15.53993994372673626, 48.99999999999997158 ) ) ;
#3076=AXIS2_PLACEMENT_3D ( 'NONE', #14779, #11621, #7782 ) ;
#3077=LINE ( 'NONE', #7906, #14951 ) ;
#3081=EDGE_CURVE ( 'NONE', #831, #6280, #4689, .T. ) ;
#3085=VECTOR ( 'NONE', #12143, 1000.000000000000000 ) ;
#3086=ORIENTED_EDGE ( 'NONE', *, *, #2167, .F. ) ;
#3087=FACE_OUTER_BOUND ( 'NONE', #6846, .T. ) ;
#3088=DIRECTION ( 'NONE',  ( 0.000000000000000000, 0.000000000000000000, -1.000000000000000000 ) ) ;
#3095=DIRECTION ( 'NONE',  ( 0.000000000000000000, -3.469446951953611033E-15, 1.000000000000000000 ) ) ;
#3097=VECTOR ( 'NONE', #7519, 1000.000000000000000 ) ;
#3099=DIRECTION ( 'NONE',  ( 1.000000000000000000, 2.751328491981765035E-32, -3.965082230804130220E-16 ) ) ;
#3108=DIRECTION ( 'NONE',  ( 0.000000000000000000, 0.000000000000000000, 1.000000000000000000 ) ) ;
#3109=CARTESIAN_POINT ( 'NONE',  ( 184.0000000000000568, 15.53993994372673981, -12.49999999999999289 ) ) ;
#3115=LINE ( 'NONE', #4057, #3744 ) ;
#3116=EDGE_LOOP ( 'NONE', ( #11301, #14275, #13967, #2775 ) ) ;
#3119=ORIENTED_EDGE ( 'NONE', *, *, #11680, .F. ) ;
#3121=CARTESIAN_POINT ( 'NONE',  ( 190.5000000000000568, -181.3058001507315566, -51.45141194869120227 ) ) ;
#3125=DIRECTION ( 'NONE',  ( -5.518327896226373923E-17, -0.9902680687415712502, -0.1391731009600586100 ) ) ;
#3126=VERTEX_POINT ( 'NONE', #11654 ) ;
#3127=CARTESIAN_POINT ( 'NONE',  ( 190.5000000000000853, -178.8058001507315566, 52.19066787724494816 ) ) ;
#3131=ORIENTED_EDGE ( 'NONE', *, *, #9496, .F. ) ;
#3133=DIRECTION ( 'NONE',  ( 0.000000000000000000, -0.9902680687415713612, 0.1391731009600582492 ) ) ;
#3134=ORIENTED_EDGE ( 'NONE', *, *, #13565, .T. ) ;
#3135=VERTEX_POINT ( 'NONE', #9133 ) ;
#3138=AXIS2_PLACEMENT_3D ( 'NONE', #3457, #5827, #10723 ) ;
#3150=( LENGTH_UNIT ( ) NAMED_UNIT ( * ) SI_UNIT ( .MILLI., .METRE. ) );
#3151=ORIENTED_EDGE ( 'NONE', *, *, #2188, .F. ) ;
#3153=CARTESIAN_POINT ( 'NONE',  ( 178.0000000000000853, -179.8058001507315566, 52.49999999999997868 ) ) ;
#3155=EDGE_CURVE ( 'NONE', #8328, #10124, #9208, .T. ) ;
#3157=ADVANCED_FACE ( 'NONE', ( #12738 ), #2162, .T. ) ;
#3158=DIRECTION ( 'NONE',  ( -3.965082230804130220E-16, 4.956352788505162775E-17, -1.000000000000000000 ) ) ;
#3159=LINE ( 'NONE', #4413, #4049 ) ;
#3167=DIRECTION ( 'NONE',  ( -0.000000000000000000, 0.000000000000000000, -1.000000000000000000 ) ) ;
#3168=EDGE_CURVE ( 'NONE', #815, #12081, #11568, .T. ) ;
#3169=AXIS2_PLACEMENT_3D ( 'NONE', #11001, #12406, #14766 ) ;
#3174=AXIS2_PLACEMENT_3D ( 'NONE', #4450, #5576, #14006 ) ;
#3175=ORIENTED_EDGE ( 'NONE', *, *, #10058, .T. ) ;
#3177=DIRECTION ( 'NONE',  ( 0.000000000000000000, -1.000000000000000000, -6.938893903907227145E-17 ) ) ;
#3178=CARTESIAN_POINT ( 'NONE',  ( 178.0000000000000853, -179.8058001507315566, 84.88378295107887084 ) ) ;
#3186=CARTESIAN_POINT ( 'NONE',  ( 184.0000000000000568, -201.3058001507315566, -42.95141194869119516 ) ) ;
#3190=ORIENTED_EDGE ( 'NONE', *, *, #10504, .T. ) ;
#3196=CARTESIAN_POINT ( 'NONE',  ( 177.5000000000000853, 15.53993994372673626, 52.49999999999997868 ) ) ;
#3197=ORIENTED_EDGE ( 'NONE', *, *, #13242, .T. ) ;
#3198=DIRECTION ( 'NONE',  ( 1.000000000000000000, -2.751328491981765035E-32, 3.965082230804130220E-16 ) ) ;
#3199=EDGE_CURVE ( 'NONE', #15193, #6271, #15179, .T. ) ;
#3201=FACE_OUTER_BOUND ( 'NONE', #2446, .T. ) ;
#3206=DIRECTION ( 'NONE',  ( -1.000000000000000000, 0.000000000000000000, 0.000000000000000000 ) ) ;
#3211=ADVANCED_FACE ( 'NONE', ( #2005 ), #13853, .F. ) ;
#3218=DIRECTION ( 'NONE',  ( 0.000000000000000000, 1.000000000000000000, 0.000000000000000000 ) ) ;
#3222=CIRCLE ( 'NONE', #7529, 0.5000000000000004441 ) ;
#3233=CIRCLE ( 'NONE', #8843, 0.5000000000000004441 ) ;
#3234=DIRECTION ( 'NONE',  ( 0.000000000000000000, 0.1391731009600660485, -0.9902680687415702510 ) ) ;
#3243=DIRECTION ( 'NONE',  ( 0.000000000000000000, 0.000000000000000000, 1.000000000000000000 ) ) ;
#3250=AXIS2_PLACEMENT_3D ( 'NONE', #4534, #15256, #2006 ) ;
#3253=CARTESIAN_POINT ( 'NONE',  ( -76.50000000000004263, -179.8058001507315566, 65.31842631998698323 ) ) ;
#3254=DIRECTION ( 'NONE',  ( 1.000000000000000000, 0.000000000000000000, 0.000000000000000000 ) ) ;
#3258=VECTOR ( 'NONE', #4124, 1000.000000000000114 ) ;
#3262=DIRECTION ( 'NONE',  ( 0.000000000000000000, 0.000000000000000000, -1.000000000000000000 ) ) ;
#3267=CIRCLE ( 'NONE', #12088, 1.499999999999994449 ) ;
#3274=VECTOR ( 'NONE', #1642, 1000.000000000000000 ) ;
#3278=CARTESIAN_POINT ( 'NONE',  ( -63.50000000000002842, 16.03993994372673626, 52.49999999999997868 ) ) ;
#3284=CIRCLE ( 'NONE', #14873, 1.500000000000001332 ) ;
#3285=DIRECTION ( 'NONE',  ( 0.000000000000000000, 0.1391731009600591096, -0.9902680687415711391 ) ) ;
#3290=DIRECTION ( 'NONE',  ( -1.000000000000000000, 0.000000000000000000, 0.000000000000000000 ) ) ;
#3292=CARTESIAN_POINT ( 'NONE',  ( -76.00000000000001421, 16.03993994372673981, -3.075184203610571654 ) ) ;
#3296=CARTESIAN_POINT ( 'NONE',  ( 190.0000000000000853, -179.8058001507315566, 52.19066787724494816 ) ) ;
#3297=CARTESIAN_POINT ( 'NONE',  ( 190.0000000000000568, -178.8058001507315566, 52.69066787724494816 ) ) ;
#3299=CIRCLE ( 'NONE', #5312, 0.4999999999999996114 ) ;
#3305=PLANE ( 'NONE',  #11687 ) ;
#3311=ORIENTED_EDGE ( 'NONE', *, *, #4911, .T. ) ;
#3313=CARTESIAN_POINT ( 'NONE',  ( 175.9483885134608272, -179.3058001507315566, 52.76585208085545275 ) ) ;
#3317=CIRCLE ( 'NONE', #12134, 0.4999999999999998890 ) ;
#3320=VERTEX_POINT ( 'NONE', #11801 ) ;
#3323=LINE ( 'NONE', #12943, #9386 ) ;
#3324=VERTEX_POINT ( 'NONE', #5955 ) ;
#3326=CIRCLE ( 'NONE', #7126, 1.499999999999994449 ) ;
#3327=CARTESIAN_POINT ( 'NONE',  ( -63.50000000000002842, -181.3058001507315566, -51.45141194869119516 ) ) ;
#3329=ORIENTED_EDGE ( 'NONE', *, *, #11650, .T. ) ;
#3333=DIRECTION ( 'NONE',  ( 1.000000000000000000, 0.000000000000000000, 0.000000000000000000 ) ) ;
#3338=EDGE_CURVE ( 'NONE', #7982, #85, #4427, .T. ) ;
#3340=AXIS2_PLACEMENT_3D ( 'NONE', #11092, #5089, #13367 ) ;
#3341=ADVANCED_FACE ( 'NONE', ( #9360 ), #13124, .T. ) ;
#3342=CLOSED_SHELL ( 'NONE', ( #11213, #3618, #12672, #6536, #14105, #15185, #8759, #4502, #15099, #14743, #14333, #5186, #5083, #2641, #12395, #1116, #5218, #9138, #8161, #14456, #4398, #5956, #2864, #6360, #13173, #2707, #12566, #4895, #12029, #15184, #13156, #10949, #11482, #5715, #9934, #7666, #10564, #417, #9754, #11415, #4597, #5464, #14352, #1417, #14875, #6632, #3353, #2281, #3341, #3024, #1344, #13864, #3074, #3157, #3500, #14125, #3632, #12248, #10826, #8770, #7606, #11467, #8849, #15064, #6651, #10683, #8129, #8943, #3421, #881, #4036, #9521, #3812, #11551, #7011, #15221 ) ) ;
#3344=VERTEX_POINT ( 'NONE', #4765 ) ;
#3345=CARTESIAN_POINT ( 'NONE',  ( 190.5000000000000853, -178.8058001507315566, 65.31842631998698323 ) ) ;
#3352=VECTOR ( 'NONE', #5067, 1000.000000000000000 ) ;
#3353=ADVANCED_FACE ( 'NONE', ( #3356 ), #9672, .T. ) ;
#3354=EDGE_CURVE ( 'NONE', #7696, #5990, #10233, .T. ) ;
#3356=FACE_OUTER_BOUND ( 'NONE', #4362, .T. ) ;
#3363=LINE ( 'NONE', #98, #2657 ) ;
#3367=DIRECTION ( 'NONE',  ( -1.000000000000000000, 0.000000000000000000, 0.000000000000000000 ) ) ;
#3369=EDGE_CURVE ( 'NONE', #2394, #14442, #15255, .T. ) ;
#3370=ORIENTED_EDGE ( 'NONE', *, *, #8761, .F. ) ;
#3371=EDGE_LOOP ( 'NONE', ( #1596, #4260, #5476, #14353 ) ) ;
#3374=CARTESIAN_POINT ( 'NONE',  ( -64.00000000000002842, 15.03993994372673804, 37.57518420361041933 ) ) ;
#3378=DIRECTION ( 'NONE',  ( 3.965082230804130220E-16, -4.956352788505162775E-17, 1.000000000000000000 ) ) ;
#3379=AXIS2_PLACEMENT_3D ( 'NONE', #4951, #15510, #8442 ) ;
#3380=DIRECTION ( 'NONE',  ( 0.000000000000000000, 0.000000000000000000, -1.000000000000000000 ) ) ;
#3384=CARTESIAN_POINT ( 'NONE',  ( -70.00000000000000000, 15.53993994372673981, -10.99999999999999645 ) ) ;
#3385=LINE ( 'NONE', #14109, #4587 ) ;
#3386=ORIENTED_EDGE ( 'NONE', *, *, #2682, .F. ) ;
#3388=SHAPE_REPRESENTATION_RELATIONSHIP ( 'NONE' , 'NONE' ,  #8648, #15417 ) ;
#3389=VERTEX_POINT ( 'NONE', #6273 ) ;
#3390=DIRECTION ( 'NONE',  ( -0.000000000000000000, 6.938893903907222067E-15, -1.000000000000000000 ) ) ;
#3401=DIRECTION ( 'NONE',  ( 0.000000000000000000, 0.000000000000000000, 1.000000000000000000 ) ) ;
#3402=EDGE_LOOP ( 'NONE', ( #9415, #8983, #583, #2926 ) ) ;
#3404=DIRECTION ( 'NONE',  ( 0.000000000000000000, 1.000000000000000000, 6.938893903907227145E-17 ) ) ;
#3408=CARTESIAN_POINT ( 'NONE',  ( -76.00000000000001421, -178.8058001507315566, 53.19066787724494816 ) ) ;
#3413=EDGE_CURVE ( 'NONE', #234, #10340, #1436, .T. ) ;
#3416=ORIENTED_EDGE ( 'NONE', *, *, #10935, .T. ) ;
#3417=CARTESIAN_POINT ( 'NONE',  ( -63.50000000000002842, 15.10952649420676863, 9.557440204760681013 ) ) ;
#3418=ORIENTED_EDGE ( 'NONE', *, *, #14970, .F. ) ;
#3419=TOROIDAL_SURFACE ( 'NONE', #5444, 1.000000000000000000, 0.5000000000000000000 ) ;
#3420=DIRECTION ( 'NONE',  ( -1.000000000000000000, 0.000000000000000000, 0.000000000000000000 ) ) ;
#3421=ADVANCED_FACE ( 'NONE', ( #12415 ), #14755, .T. ) ;
#3431=DIRECTION ( 'NONE',  ( -5.518327896226373923E-17, 0.9902680687415712502, 0.1391731009600586100 ) ) ;
#3438=CARTESIAN_POINT ( 'NONE',  ( 190.5000000000000568, -178.7362136002515172, -17.68580191161595394 ) ) ;
#3442=EDGE_CURVE ( 'NONE', #14585, #12671, #14624, .T. ) ;
#3449=ORIENTED_EDGE ( 'NONE', *, *, #11312, .T. ) ;
#3452=LINE ( 'NONE', #12836, #8924 ) ;
#3453=CARTESIAN_POINT ( 'NONE',  ( -76.50000000000004263, -178.9449732516916072, 64.32815825124538378 ) ) ;
#3457=CARTESIAN_POINT ( 'NONE',  ( -64.00000000000002842, 16.03993994372673981, 7.553451883674125344E-16 ) ) ;
#3460=DIRECTION ( 'NONE',  ( 0.000000000000000000, 0.000000000000000000, 1.000000000000000000 ) ) ;
#3461=ORIENTED_EDGE ( 'NONE', *, *, #4189, .F. ) ;
#3464=DIRECTION ( 'NONE',  ( 0.000000000000000000, 0.1391731009600660485, -0.9902680687415702510 ) ) ;
#3465=CARTESIAN_POINT ( 'NONE',  ( -70.00000000000000000, -201.3058001507315566, -42.95141194869119516 ) ) ;
#3468=ORIENTED_EDGE ( 'NONE', *, *, #13150, .F. ) ;
#3477=ORIENTED_EDGE ( 'NONE', *, *, #455, .F. ) ;
#3478=VERTEX_POINT ( 'NONE', #3967 ) ;
#3480=DIRECTION ( 'NONE',  ( -0.000000000000000000, -4.956352788505162775E-17, 1.000000000000000000 ) ) ;
#3481=ORIENTED_EDGE ( 'NONE', *, *, #10450, .F. ) ;
#3486=EDGE_CURVE ( 'NONE', #7029, #13870, #4163, .T. ) ;
#3488=VERTEX_POINT ( 'NONE', #7538 ) ;
#3490=LINE ( 'NONE', #15399, #12841 ) ;
#3500=ADVANCED_FACE ( 'NONE', ( #91 ), #3419, .T. ) ;
#3504=CARTESIAN_POINT ( 'NONE',  ( 184.0000000000000568, -181.3058001507315566, -41.45141194869120227 ) ) ;
#3507=AXIS2_PLACEMENT_3D ( 'NONE', #884, #9202, #9276 ) ;
#3514=DIRECTION ( 'NONE',  ( 1.077120774387149835E-15, -0.9902680687415711391, 0.1391731009600592484 ) ) ;
#3515=LINE ( 'NONE', #2250, #8965 ) ;
#3519=FACE_OUTER_BOUND ( 'NONE', #9583, .T. ) ;
#3523=CARTESIAN_POINT ( 'NONE',  ( -76.50000000000001421, -179.8058001507315566, -17.19066787724516843 ) ) ;
#3526=DIRECTION ( 'NONE',  ( -1.000000000000000000, 0.000000000000000000, 0.000000000000000000 ) ) ;
#3527=DIRECTION ( 'NONE',  ( 0.000000000000000000, 0.000000000000000000, -1.000000000000000000 ) ) ;
#3528=CIRCLE ( 'NONE', #2778, 0.4999999999999998890 ) ;
#3530=AXIS2_PLACEMENT_3D ( 'NONE', #13518, #8724, #9993 ) ;
#3535=AXIS2_PLACEMENT_3D ( 'NONE', #12958, #1986, #9195 ) ;
#3537=EDGE_CURVE ( 'NONE', #5369, #15306, #8961, .T. ) ;
#3539=DIRECTION ( 'NONE',  ( 0.000000000000000000, 2.775557561562888827E-14, 1.000000000000000000 ) ) ;
#3544=CARTESIAN_POINT ( 'NONE',  ( 190.0000000000000853, 15.17911304468679745, 25.93769382960994818 ) ) ;
#3547=DIRECTION ( 'NONE',  ( -1.000000000000000000, 0.000000000000000000, 0.000000000000000000 ) ) ;
#3551=AXIS2_PLACEMENT_3D ( 'NONE', #6958, #854, #8069 ) ;
#3553=VECTOR ( 'NONE', #3927, 1000.000000000000000 ) ;
#3556=FACE_OUTER_BOUND ( 'NONE', #14843, .T. ) ;
#3557=ORIENTED_EDGE ( 'NONE', *, *, #1390, .F. ) ;
#3561=VERTEX_POINT ( 'NONE', #640 ) ;
#3566=ORIENTED_EDGE ( 'NONE', *, *, #13771, .F. ) ;
#3568=CARTESIAN_POINT ( 'NONE',  ( 190.0000000000000568, 16.03993994372673981, 10.05257423913146475 ) ) ;
#3571=VERTEX_POINT ( 'NONE', #15009 ) ;
#3572=ORIENTED_EDGE ( 'NONE', *, *, #7804, .F. ) ;
#3574=ORIENTED_EDGE ( 'NONE', *, *, #7254, .F. ) ;
#3577=EDGE_CURVE ( 'NONE', #6971, #7619, #13751, .T. ) ;
#3579=ORIENTED_EDGE ( 'NONE', *, *, #3920, .T. ) ;
#3586=EDGE_CURVE ( 'NONE', #11697, #12019, #9247, .T. ) ;
#3587=DIRECTION ( 'NONE',  ( 0.000000000000000000, 0.1391731009600584990, -0.9902680687415712502 ) ) ;
#3590=ORIENTED_EDGE ( 'NONE', *, *, #1602, .T. ) ;
#3592=CARTESIAN_POINT ( 'NONE',  ( 177.5000000000000853, 17.53993994372673981, -17.50000000000002487 ) ) ;
#3594=EDGE_LOOP ( 'NONE', ( #1330, #13326, #7221, #14882 ) ) ;
#3595=FACE_OUTER_BOUND ( 'NONE', #4043, .T. ) ;
#3596=DIRECTION ( 'NONE',  ( 0.000000000000000000, 0.9902680687415702510, 0.1391731009600660485 ) ) ;
#3598=DIRECTION ( 'NONE',  ( 0.000000000000000000, 0.000000000000000000, -1.000000000000000000 ) ) ;
#3604=VERTEX_POINT ( 'NONE', #13832 ) ;
#3606=LINE ( 'NONE', #10637, #11600 ) ;
#3611=VECTOR ( 'NONE', #3378, 1000.000000000000000 ) ;
#3616=DIRECTION ( 'NONE',  ( 0.000000000000000000, 0.000000000000000000, -1.000000000000000000 ) ) ;
#3618=ADVANCED_FACE ( 'NONE', ( #476 ), #1680, .F. ) ;
#3620=DIRECTION ( 'NONE',  ( -1.000000000000000000, -0.000000000000000000, -0.000000000000000000 ) ) ;
#3622=VECTOR ( 'NONE', #11031, 1000.000000000000000 ) ;
#3624=LINE ( 'NONE', #2677, #8665 ) ;
#3628=ORIENTED_EDGE ( 'NONE', *, *, #3413, .T. ) ;
#3629=ORIENTED_EDGE ( 'NONE', *, *, #3442, .T. ) ;
#3631=ORIENTED_EDGE ( 'NONE', *, *, #9662, .F. ) ;
#3632=ADVANCED_FACE ( 'NONE', ( #12647 ), #13917, .F. ) ;
#3635=EDGE_CURVE ( 'NONE', #8082, #3571, #11315, .T. ) ;
#3637=ORIENTED_EDGE ( 'NONE', *, *, #6614, .T. ) ;
#3639=LINE ( 'NONE', #7796, #3988 ) ;
#3640=LINE ( 'NONE', #2381, #9118 ) ;
#3643=CARTESIAN_POINT ( 'NONE',  ( -63.50000000000002842, -179.3058001507315566, 65.31842631998698323 ) ) ;
#3650=CIRCLE ( 'NONE', #8213, 1.000000000000000888 ) ;
#3661=AXIS2_PLACEMENT_3D ( 'NONE', #2390, #11950, #3420 ) ;
#3664=EDGE_CURVE ( 'NONE', #10667, #3488, #12798, .T. ) ;
#3671=CARTESIAN_POINT ( 'NONE',  ( 178.0000000000000853, 21.51947656765318229, 9.953386152224130257 ) ) ;
#3676=ORIENTED_EDGE ( 'NONE', *, *, #7183, .F. ) ;
#3679=AXIS2_PLACEMENT_3D ( 'NONE', #6438, #398, #6357 ) ;
#3681=DIRECTION ( 'NONE',  ( -0.000000000000000000, -0.9902680687415712502, -0.1391731009600586100 ) ) ;
#3685=AXIS2_PLACEMENT_3D ( 'NONE', #10140, #6086, #128 ) ;
#3686=DIRECTION ( 'NONE',  ( -0.000000000000000000, 0.9902680687415713612, -0.1391731009600582492 ) ) ;
#3687=CIRCLE ( 'NONE', #11259, 0.5000000000000004441 ) ;
#3689=CARTESIAN_POINT ( 'NONE',  ( 177.5000000000000853, -179.3753867012115961, -29.38864891670827362 ) ) ;
#3691=ADVANCED_FACE ( 'NONE', ( #9268 ), #1667, .T. ) ;
#3694=ORIENTED_EDGE ( 'NONE', *, *, #14509, .F. ) ;
#3695=DIRECTION ( 'NONE',  ( -1.000000000000000000, 0.000000000000000000, 0.000000000000000000 ) ) ;
#3696=CARTESIAN_POINT ( 'NONE',  ( -70.00000000000000000, 15.53993994372673626, 47.49999999999997868 ) ) ;
#3698=( LENGTH_UNIT ( ) NAMED_UNIT ( * ) SI_UNIT ( .MILLI., .METRE. ) );
#3701=AXIS2_PLACEMENT_3D ( 'NONE', #5840, #13402, #2600 ) ;
#3704=VERTEX_POINT ( 'NONE', #12223 ) ;
#3705=EDGE_CURVE ( 'NONE', #12666, #13605, #5710, .T. ) ;
#3708=DIRECTION ( 'NONE',  ( -1.000000000000000000, 0.000000000000000000, 0.000000000000000000 ) ) ;
#3716=DIRECTION ( 'NONE',  ( 0.000000000000000000, 0.000000000000000000, -1.000000000000000000 ) ) ;
#3720=CIRCLE ( 'NONE', #3973, 0.5000000000000004441 ) ;
#3725=ADVANCED_FACE ( 'NONE', ( #8096 ), #12071, .F. ) ;
#3726=CARTESIAN_POINT ( 'NONE',  ( 177.5000000000000853, 15.17911304468679745, 25.93769382960995884 ) ) ;
#3728=DIRECTION ( 'NONE',  ( 0.000000000000000000, 0.000000000000000000, -1.000000000000000000 ) ) ;
#3735=CIRCLE ( 'NONE', #7030, 0.4999999999999996114 ) ;
#3738=DIRECTION ( 'NONE',  ( -5.518327896226369609E-17, -0.9902680687415712502, -0.1391731009600584990 ) ) ;
#3741=AXIS2_PLACEMENT_3D ( 'NONE', #4266, #11780, #946 ) ;
#3742=EDGE_LOOP ( 'NONE', ( #9867, #8103, #13264, #5637, #1035 ) ) ;
#3744=VECTOR ( 'NONE', #4132, 1000.000000000000000 ) ;
#3747=ORIENTED_EDGE ( 'NONE', *, *, #7881, .T. ) ;
#3750=EDGE_CURVE ( 'NONE', #9812, #15306, #9801, .T. ) ;
#3756=VERTEX_POINT ( 'NONE', #14432 ) ;
#3757=ORIENTED_EDGE ( 'NONE', *, *, #6516, .F. ) ;
#3760=LINE ( 'NONE', #4193, #7841 ) ;
#3763=DIRECTION ( 'NONE',  ( 0.000000000000000000, 0.000000000000000000, -1.000000000000000000 ) ) ;
#3764=DIRECTION ( 'NONE',  ( 1.000000000000000000, -0.000000000000000000, -0.000000000000000000 ) ) ;
#3771=DIRECTION ( 'NONE',  ( -0.000000000000000000, 1.000000000000000000, 6.938893903907227145E-17 ) ) ;
#3774=AXIS2_PLACEMENT_3D ( 'NONE', #423, #1858, #1705 ) ;
#3776=CARTESIAN_POINT ( 'NONE',  ( 177.5000000000000853, 15.53993994372673981, -17.50000000000002487 ) ) ;
#3777=VECTOR ( 'NONE', #12339, 1000.000000000000000 ) ;
#3780=DIRECTION ( 'NONE',  ( 0.000000000000000000, -1.000000000000000000, -4.956352788505160310E-17 ) ) ;
#3783=CIRCLE ( 'NONE', #5797, 1.500000000000001332 ) ;
#3784=CARTESIAN_POINT ( 'NONE',  ( -64.00000000000002842, -178.8058001507315566, 65.31842631998698323 ) ) ;
#3788=AXIS2_PLACEMENT_3D ( 'NONE', #6789, #4405, #11441 ) ;
#3793=VERTEX_POINT ( 'NONE', #10052 ) ;
#3796=CARTESIAN_POINT ( 'NONE',  ( 178.0000000000000853, 15.53993994372673981, 9.617930870223348805 ) ) ;
#3798=EDGE_CURVE ( 'NONE', #10971, #2355, #13054, .T. ) ;
#3800=CARTESIAN_POINT ( 'NONE',  ( 178.0000000000000853, -178.8058001507315566, -30.31842631998718574 ) ) ;
#3802=VECTOR ( 'NONE', #15060, 1000.000000000000000 ) ;
#3812=ADVANCED_FACE ( 'NONE', ( #7768 ), #1720, .T. ) ;
#3814=VECTOR ( 'NONE', #7172, 1000.000000000000000 ) ;
#3822=DIRECTION ( 'NONE',  ( 1.000000000000000000, -2.751328491981765035E-32, 3.965082230804130220E-16 ) ) ;
#3824=EDGE_CURVE ( 'NONE', #8794, #944, #13667, .T. ) ;
#3826=LINE ( 'NONE', #8646, #11079 ) ;
#3828=CIRCLE ( 'NONE', #3076, 0.5000000000000000000 ) ;
#3829=VERTEX_POINT ( 'NONE', #1749 ) ;
#3830=CARTESIAN_POINT ( 'NONE',  ( -76.00000000000001421, -178.8058001507315566, 52.69066787724494816 ) ) ;
#3832=VERTEX_POINT ( 'NONE', #11307 ) ;
#3838=CIRCLE ( 'NONE', #5853, 1.000000000000000888 ) ;
#3840=EDGE_CURVE ( 'NONE', #12019, #3756, #468, .T. ) ;
#3845=AXIS2_PLACEMENT_3D ( 'NONE', #5679, #3460, #7106 ) ;
#3849=DIRECTION ( 'NONE',  ( 0.000000000000000000, -0.9902680687415712502, -0.1391731009600586100 ) ) ;
#3854=CARTESIAN_POINT ( 'NONE',  ( -76.00000000000004263, -179.3058001507315566, 64.88378295107887084 ) ) ;
#3857=DIRECTION ( 'NONE',  ( 0.000000000000000000, -0.1391731009600641333, -0.9902680687415704730 ) ) ;
#3862=CARTESIAN_POINT ( 'NONE',  ( -76.00000000000001421, 15.03993994372673981, -3.075184203610571654 ) ) ;
#3865=ORIENTED_EDGE ( 'NONE', *, *, #1797, .T. ) ;
#3866=CIRCLE ( 'NONE', #12673, 0.5000000000000004441 ) ;
#3867=EDGE_CURVE ( 'NONE', #8197, #3324, #8716, .T. ) ;
#3878=DIRECTION ( 'NONE',  ( 0.000000000000000000, -0.9902680687415712502, -0.1391731009600596092 ) ) ;
#3882=EDGE_LOOP ( 'NONE', ( #5039, #5265 ) ) ;
#3885=ORIENTED_EDGE ( 'NONE', *, *, #13530, .F. ) ;
#3886=CIRCLE ( 'NONE', #840, 1.000000000000000888 ) ;
#3887=CARTESIAN_POINT ( 'NONE',  ( -76.00000000000001421, 15.53993994372673981, 10.05257423913146475 ) ) ;
#3890=CARTESIAN_POINT ( 'NONE',  ( 184.0000000000000568, -181.3058001507315566, 77.95141194869098911 ) ) ;
#3891=ORIENTED_EDGE ( 'NONE', *, *, #1198, .T. ) ;
#3893=DIRECTION ( 'NONE',  ( -1.000000000000000000, 0.000000000000000000, 0.000000000000000000 ) ) ;
#3894=EDGE_CURVE ( 'NONE', #5784, #10772, #9051, .T. ) ;
#3898=CARTESIAN_POINT ( 'NONE',  ( -64.00000000000002842, -178.9449732516916072, -29.32815825124560760 ) ) ;
#3912=ORIENTED_EDGE ( 'NONE', *, *, #13958, .T. ) ;
#3915=FACE_OUTER_BOUND ( 'NONE', #8848, .T. ) ;
#3920=EDGE_CURVE ( 'NONE', #8640, #4430, #13567, .T. ) ;
#3921=DIRECTION ( 'NONE',  ( 1.000000000000000000, 0.000000000000000000, 3.965082230804112963E-16 ) ) ;
#3927=DIRECTION ( 'NONE',  ( 5.518327896226373923E-17, -0.9902680687415712502, -0.1391731009600586100 ) ) ;
#3928=EDGE_LOOP ( 'NONE', ( #7060, #121, #6529, #3566 ) ) ;
#3934=DIRECTION ( 'NONE',  ( -1.000000000000000000, 0.000000000000000000, 0.000000000000000000 ) ) ;
#3940=DIRECTION ( 'NONE',  ( 0.000000000000000000, 1.000000000000000000, 6.938893903907227145E-17 ) ) ;
#3950=FACE_OUTER_BOUND ( 'NONE', #5492, .T. ) ;
#3953=DIRECTION ( 'NONE',  ( 0.000000000000000000, -0.1391731009600660485, -0.9902680687415702510 ) ) ;
#3965=EDGE_CURVE ( 'NONE', #6346, #9678, #9263, .T. ) ;
#3967=CARTESIAN_POINT ( 'NONE',  ( -63.50000000000002842, -179.8058001507315566, 65.31842631998698323 ) ) ;
#3973=AXIS2_PLACEMENT_3D ( 'NONE', #2941, #4112, #3016 ) ;
#3982=DIRECTION ( 'NONE',  ( -0.000000000000000000, 1.000000000000000000, 6.938893903907227145E-17 ) ) ;
#3983=PLANE ( 'NONE',  #6478 ) ;
#3985=VECTOR ( 'NONE', #11034, 1000.000000000000000 ) ;
#3988=VECTOR ( 'NONE', #9491, 1000.000000000000000 ) ;
#3992=DIRECTION ( 'NONE',  ( 0.000000000000000000, 1.000000000000000000, 6.938893903907222067E-15 ) ) ;
#3994=EDGE_CURVE ( 'NONE', #10853, #5266, #6774, .T. ) ;
#4001=CARTESIAN_POINT ( 'NONE',  ( -70.00000000000000000, -181.3058001507315566, 76.45141194869098911 ) ) ;
#4008=EDGE_CURVE ( 'NONE', #5990, #3704, #8784, .T. ) ;
#4010=CIRCLE ( 'NONE', #3009, 0.5000000000000004441 ) ;
#4018=ORIENTED_EDGE ( 'NONE', *, *, #9853, .F. ) ;
#4020=DIRECTION ( 'NONE',  ( 0.000000000000000000, -1.000000000000000000, 0.000000000000000000 ) ) ;
#4026=CARTESIAN_POINT ( 'NONE',  ( 190.0000000000000568, 11.87216911405867670, 8.597545510065431884 ) ) ;
#4028=VERTEX_POINT ( 'NONE', #703 ) ;
#4029=TOROIDAL_SURFACE ( 'NONE', #5564, 1.000000000000000000, 0.5000000000000000000 ) ;
#4036=ADVANCED_FACE ( 'NONE', ( #11628 ), #15390, .F. ) ;
#4043=EDGE_LOOP ( 'NONE', ( #6956, #15068, #3151, #3747, #7627, #11912 ) ) ;
#4048=DIRECTION ( 'NONE',  ( 0.000000000000000000, -1.000000000000000000, 0.000000000000000000 ) ) ;
#4049=VECTOR ( 'NONE', #7915, 1000.000000000000000 ) ;
#4051=PRESENTATION_STYLE_ASSIGNMENT (( #11173 ) ) ;
#4052=EDGE_CURVE ( 'NONE', #15155, #8082, #15316, .T. ) ;
#4057=CARTESIAN_POINT ( 'NONE',  ( -76.50000000000004263, 15.53993994372673626, 52.49999999999997868 ) ) ;
#4064=DIRECTION ( 'NONE',  ( 1.000000000000000000, 0.000000000000000000, 0.000000000000000000 ) ) ;
#4065=CARTESIAN_POINT ( 'NONE',  ( 184.0000000000000568, 15.53993994372673981, -10.99999999999999645 ) ) ;
#4069=CARTESIAN_POINT ( 'NONE',  ( -61.94838851346079167, -179.3058001507315566, -17.76585208085566947 ) ) ;
#4071=VECTOR ( 'NONE', #12530, 1000.000000000000000 ) ;
#4074=CYLINDRICAL_SURFACE ( 'NONE', #5253, 1.499999999999997780 ) ;
#4079=CARTESIAN_POINT ( 'NONE',  ( -64.00000000000002842, 15.53993994372673804, 24.94742576086838781 ) ) ;
#4084=EDGE_CURVE ( 'NONE', #12187, #5228, #3639, .T. ) ;
#4088=VECTOR ( 'NONE', #4540, 1000.000000000000000 ) ;
#4091=EDGE_LOOP ( 'NONE', ( #15037, #1289, #793, #15522 ) ) ;
#4093=EDGE_CURVE ( 'NONE', #13859, #12311, #12012, .T. ) ;
#4098=ORIENTED_EDGE ( 'NONE', *, *, #436, .F. ) ;
#4111=EDGE_CURVE ( 'NONE', #10853, #8004, #4740, .T. ) ;
#4112=DIRECTION ( 'NONE',  ( 1.000000000000000000, 2.751328491981765035E-32, -3.965082230804130220E-16 ) ) ;
#4113=ORIENTED_EDGE ( 'NONE', *, *, #5152, .F. ) ;
#4115=DIRECTION ( 'NONE',  ( 0.000000000000000000, 0.000000000000000000, 1.000000000000000000 ) ) ;
#4116=ORIENTED_EDGE ( 'NONE', *, *, #14690, .F. ) ;
#4123=AXIS2_PLACEMENT_3D ( 'NONE', #14874, #6458, #5106 ) ;
#4124=DIRECTION ( 'NONE',  ( 0.000000000000000000, 0.9902680687415713612, -0.1391731009600582492 ) ) ;
#4125=DIRECTION ( 'NONE',  ( -1.000000000000000000, 0.000000000000000000, 0.000000000000000000 ) ) ;
#4126=DIRECTION ( 'NONE',  ( 0.000000000000000000, 1.000000000000000000, -0.000000000000000000 ) ) ;
#4129=ORIENTED_EDGE ( 'NONE', *, *, #13754, .F. ) ;
#4130=CARTESIAN_POINT ( 'NONE',  ( 190.5000000000000568, 17.53993994372673981, -17.50000000000002487 ) ) ;
#4132=DIRECTION ( 'NONE',  ( 1.000000000000000000, 0.000000000000000000, 0.000000000000000000 ) ) ;
#4133=ORIENTED_EDGE ( 'NONE', *, *, #14190, .T. ) ;
#4147=CARTESIAN_POINT ( 'NONE',  ( 184.0000000000000568, -179.3058001507315566, -41.45141194869120227 ) ) ;
#4154=LINE ( 'NONE', #7736, #15436 ) ;
#4155=DIRECTION ( 'NONE',  ( 0.000000000000000000, -1.000000000000000000, 0.000000000000000000 ) ) ;
#4160=CIRCLE ( 'NONE', #7462, 1.000000000000000888 ) ;
#4163=CIRCLE ( 'NONE', #7463, 0.4999999999999996114 ) ;
#4169=VERTEX_POINT ( 'NONE', #11859 ) ;
#4176=EDGE_CURVE ( 'NONE', #6305, #7344, #4909, .T. ) ;
#4184=CARTESIAN_POINT ( 'NONE',  ( 177.5000000000000853, -178.8058001507315566, -17.19066787724516843 ) ) ;
#4187=ORIENTED_EDGE ( 'NONE', *, *, #9421, .F. ) ;
#4189=EDGE_CURVE ( 'NONE', #13452, #12639, #10914, .T. ) ;
#4190=DIRECTION ( 'NONE',  ( 0.000000000000000000, -0.1391731009600641333, -0.9902680687415704730 ) ) ;
#4193=CARTESIAN_POINT ( 'NONE',  ( -76.00000000000001421, -179.3058001507315282, -29.88378295107906268 ) ) ;
#4196=EDGE_CURVE ( 'NONE', #227, #6305, #2380, .T. ) ;
#4197=EDGE_CURVE ( 'NONE', #13871, #12666, #9815, .T. ) ;
#4200=DIRECTION ( 'NONE',  ( 0.000000000000000000, 0.000000000000000000, -1.000000000000000000 ) ) ;
#4202=DIRECTION ( 'NONE',  ( 3.965082230804130220E-16, 0.000000000000000000, 1.000000000000000000 ) ) ;
#4212=CARTESIAN_POINT ( 'NONE',  ( -76.00000000000001421, -179.8058001507315566, -51.45141194869120937 ) ) ;
#4213=DIRECTION ( 'NONE',  ( 0.000000000000000000, 0.000000000000000000, -1.000000000000000000 ) ) ;
#4214=EDGE_CURVE ( 'NONE', #5867, #12589, #14596, .T. ) ;
#4220=DIRECTION ( 'NONE',  ( 0.000000000000000000, 0.000000000000000000, 1.000000000000000000 ) ) ;
#4222=DIRECTION ( 'NONE',  ( -0.000000000000000000, -0.000000000000000000, 1.000000000000000000 ) ) ;
#4225=CARTESIAN_POINT ( 'NONE',  ( -76.50000000000001421, -179.3058001507315566, 52.19066787724494816 ) ) ;
#4226=EDGE_CURVE ( 'NONE', #3135, #3829, #296, .T. ) ;
#4227=AXIS2_PLACEMENT_3D ( 'NONE', #13710, #2914, #14660 ) ;
#4228=ORIENTED_EDGE ( 'NONE', *, *, #10592, .F. ) ;
#4235=CARTESIAN_POINT ( 'NONE',  ( -70.00000000000000000, 15.53993994372673981, -12.49999999999999289 ) ) ;
#4236=DIRECTION ( 'NONE',  ( 0.000000000000000000, 0.000000000000000000, 1.000000000000000000 ) ) ;
#4238=CARTESIAN_POINT ( 'NONE',  ( -76.50000000000001421, 15.17911304468679923, 9.062306170389897275 ) ) ;
#4239=PLANE ( 'NONE',  #1099 ) ;
#4240=AXIS2_PLACEMENT_3D ( 'NONE', #13926, #8893, #15093 ) ;
#4241=DIRECTION ( 'NONE',  ( 0.000000000000000000, 0.000000000000000000, 1.000000000000000000 ) ) ;
#4242=CARTESIAN_POINT ( 'NONE',  ( -76.00000000000001421, 15.53993994372673804, 24.94742576086838781 ) ) ;
#4245=ORIENTED_EDGE ( 'NONE', *, *, #10393, .F. ) ;
#4247=CARTESIAN_POINT ( 'NONE',  ( 190.0000000000000568, 15.53993994372673981, -17.50000000000002487 ) ) ;
#4251=CIRCLE ( 'NONE', #1990, 0.5000000000000004441 ) ;
#4256=ORIENTED_EDGE ( 'NONE', *, *, #13041, .T. ) ;
#4257=AXIS2_PLACEMENT_3D ( 'NONE', #2399, #3822, #1520 ) ;
#4259=CARTESIAN_POINT ( 'NONE',  ( -76.50000000000004263, -178.8058001507315566, 52.19066787724494816 ) ) ;
#4260=ORIENTED_EDGE ( 'NONE', *, *, #13091, .T. ) ;
#4265=EDGE_LOOP ( 'NONE', ( #9334, #11185 ) ) ;
#4266=CARTESIAN_POINT ( 'NONE',  ( 175.9483885134608272, -178.8058001507315566, -30.31842631998718574 ) ) ;
#4275=DIRECTION ( 'NONE',  ( 0.000000000000000000, 1.000000000000000000, 0.000000000000000000 ) ) ;
#4279=CIRCLE ( 'NONE', #13107, 0.5000000000000004441 ) ;
#4280=ORIENTED_EDGE ( 'NONE', *, *, #2663, .T. ) ;
#4281=DIRECTION ( 'NONE',  ( 1.000000000000000000, -2.751328491981765035E-32, 3.965082230804130220E-16 ) ) ;
#4282=VECTOR ( 'NONE', #1304, 1000.000000000000000 ) ;
#4290=VERTEX_POINT ( 'NONE', #15286 ) ;
#4296=AXIS2_PLACEMENT_3D ( 'NONE', #13269, #9353, #961 ) ;
#4307=CIRCLE ( 'NONE', #14390, 1.499999999999994449 ) ;
#4309=ORIENTED_EDGE ( 'NONE', *, *, #11257, .T. ) ;
#4310=ORIENTED_EDGE ( 'NONE', *, *, #10324, .T. ) ;
#4313=DIRECTION ( 'NONE',  ( 2.751328491981765035E-32, -1.000000000000000000, -1.090924371466202084E-47 ) ) ;
#4315=DIRECTION ( 'NONE',  ( 0.000000000000000000, 0.000000000000000000, -1.000000000000000000 ) ) ;
#4318=CIRCLE ( 'NONE', #268, 0.5000000000000004441 ) ;
#4319=EDGE_CURVE ( 'NONE', #620, #12599, #4505, .T. ) ;
#4320=CARTESIAN_POINT ( 'NONE',  ( 178.0000000000000853, -179.3058001507315566, 52.19066787724494816 ) ) ;
#4326=VERTEX_POINT ( 'NONE', #7986 ) ;
#4333=FACE_OUTER_BOUND ( 'NONE', #5757, .T. ) ;
#4336=ADVANCED_FACE ( 'NONE', ( #7834 ), #2759, .T. ) ;
#4338=CARTESIAN_POINT ( 'NONE',  ( -70.00000000000000000, -181.3058001507315566, -41.45141194869120227 ) ) ;
#4339=ORIENTED_EDGE ( 'NONE', *, *, #7881, .F. ) ;
#4344=ORIENTED_EDGE ( 'NONE', *, *, #13204, .T. ) ;
#4347=PLANE ( 'NONE',  #7726 ) ;
#4348=FACE_OUTER_BOUND ( 'NONE', #12072, .T. ) ;
#4349=ORIENTED_EDGE ( 'NONE', *, *, #804, .F. ) ;
#4351=DIRECTION ( 'NONE',  ( -0.000000000000000000, 0.9902680687415702510, -0.1391731009600660485 ) ) ;
#4352=LINE ( 'NONE', #9264, #15392 ) ;
#4353=EDGE_LOOP ( 'NONE', ( #11819, #8906, #11787, #8967 ) ) ;
#4356=DIRECTION ( 'NONE',  ( 1.000000000000000000, 0.000000000000000000, 0.000000000000000000 ) ) ;
#4362=EDGE_LOOP ( 'NONE', ( #8628, #1491, #6705, #10705 ) ) ;
#4364=DIRECTION ( 'NONE',  ( 3.965082230804130220E-16, -4.956352788505162775E-17, 1.000000000000000000 ) ) ;
#4366=FACE_OUTER_BOUND ( 'NONE', #6041, .T. ) ;
#4375=DIRECTION ( 'NONE',  ( 0.000000000000000000, -1.000000000000000000, 0.000000000000000000 ) ) ;
#4382=CARTESIAN_POINT ( 'NONE',  ( 190.0000000000000568, 15.03993994372673981, -2.075184203610571210 ) ) ;
#4383=AXIS2_PLACEMENT_3D ( 'NONE', #8857, #1577, #12467 ) ;
#4388=DIRECTION ( 'NONE',  ( 0.000000000000000000, 0.000000000000000000, 1.000000000000000000 ) ) ;
#4389=VERTEX_POINT ( 'NONE', #5450 ) ;
#4392=CARTESIAN_POINT ( 'NONE',  ( -64.00000000000002842, 14.90076684276667862, 37.08491613486885541 ) ) ;
#4397=ADVANCED_FACE ( 'NONE', ( #8064, #4484 ), #928, .T. ) ;
#4398=ADVANCED_FACE ( 'NONE', ( #2040 ), #6876, .T. ) ;
#4399=EDGE_CURVE ( 'NONE', #13797, #14752, #12322, .T. ) ;
#4402=EDGE_CURVE ( 'NONE', #5220, #3389, #13834, .T. ) ;
#4405=DIRECTION ( 'NONE',  ( -1.000000000000000000, 0.000000000000000000, 0.000000000000000000 ) ) ;
#4407=ORIENTED_EDGE ( 'NONE', *, *, #5524, .T. ) ;
#4411=ORIENTED_EDGE ( 'NONE', *, *, #9191, .F. ) ;
#4412=PRESENTATION_STYLE_ASSIGNMENT (( #12935 ) ) ;
#4413=CARTESIAN_POINT ( 'NONE',  ( 184.0000000000000568, 15.53993994372673981, -10.99999999999999645 ) ) ;
#4414=CIRCLE ( 'NONE', #8474, 1.499999999999997780 ) ;
#4415=CARTESIAN_POINT ( 'NONE',  ( 190.0000000000000568, -178.6666270497714777, -18.18093594598673945 ) ) ;
#4416=ORIENTED_EDGE ( 'NONE', *, *, #14190, .F. ) ;
#4420=ORIENTED_EDGE ( 'NONE', *, *, #2378, .F. ) ;
#4423=CARTESIAN_POINT ( 'NONE',  ( 190.0000000000000568, 16.03993994372673981, -3.075184203610571654 ) ) ;
#4425=EDGE_LOOP ( 'NONE', ( #13324, #13214, #10783, #11081 ) ) ;
#4427=CIRCLE ( 'NONE', #15003, 1.499999999999994449 ) ;
#4430=VERTEX_POINT ( 'NONE', #14499 ) ;
#4431=CARTESIAN_POINT ( 'NONE',  ( 178.0000000000000853, -179.8058001507315566, -51.45141194869119516 ) ) ;
#4436=VECTOR ( 'NONE', #10449, 1000.000000000000000 ) ;
#4442=CYLINDRICAL_SURFACE ( 'NONE', #5278, 0.5000000000000004441 ) ;
#4443=ORIENTED_EDGE ( 'NONE', *, *, #12145, .F. ) ;
#4444=EDGE_CURVE ( 'NONE', #4326, #6739, #4251, .T. ) ;
#4447=VERTEX_POINT ( 'NONE', #9628 ) ;
#4448=CIRCLE ( 'NONE', #15024, 1.500000000000001332 ) ;
#4450=CARTESIAN_POINT ( 'NONE',  ( -76.00000000000001421, 15.03993994372673981, 10.05257423913146475 ) ) ;
#4451=DIRECTION ( 'NONE',  ( -9.657073818396194363E-16, 0.9902680687415711391, -0.1391731009600592484 ) ) ;
#4452=ORIENTED_EDGE ( 'NONE', *, *, #3486, .T. ) ;
#4455=VECTOR ( 'NONE', #7580, 1000.000000000000000 ) ;
#4460=DIRECTION ( 'NONE',  ( 0.000000000000000000, 0.1391731009600626345, 0.9902680687415706950 ) ) ;
#4461=ORIENTED_EDGE ( 'NONE', *, *, #6359, .F. ) ;
#4464=ORIENTED_EDGE ( 'NONE', *, *, #4578, .T. ) ;
#4472=LINE ( 'NONE', #3075, #67 ) ;
#4476=CIRCLE ( 'NONE', #2982, 0.5000000000000004441 ) ;
#4481=( NAMED_UNIT ( * ) PLANE_ANGLE_UNIT ( ) SI_UNIT ( $, .RADIAN. ) );
#4482=EDGE_CURVE ( 'NONE', #14401, #14171, #5497, .T. ) ;
#4484=FACE_BOUND ( 'NONE', #9542, .T. ) ;
#4486=ORIENTED_EDGE ( 'NONE', *, *, #4402, .T. ) ;
#4492=DIRECTION ( 'NONE',  ( -0.000000000000000000, -0.000000000000000000, -1.000000000000000000 ) ) ;
#4493=ORIENTED_EDGE ( 'NONE', *, *, #7219, .F. ) ;
#4497=CYLINDRICAL_SURFACE ( 'NONE', #5343, 0.5000000000000004441 ) ;
#4498=ORIENTED_EDGE ( 'NONE', *, *, #15382, .F. ) ;
#4499=FACE_OUTER_BOUND ( 'NONE', #12241, .T. ) ;
#4501=DIRECTION ( 'NONE',  ( 0.000000000000000000, 6.938893903907227145E-17, -1.000000000000000000 ) ) ;
#4502=ADVANCED_FACE ( 'NONE', ( #14344 ), #8316, .T. ) ;
#4504=EDGE_LOOP ( 'NONE', ( #572, #5833, #4653, #5365 ) ) ;
#4505=CIRCLE ( 'NONE', #7808, 0.5000000000000004441 ) ;
#4506=ORIENTED_EDGE ( 'NONE', *, *, #10101, .T. ) ;
#4508=CARTESIAN_POINT ( 'NONE',  ( 190.5000000000000568, 15.47035339324671099, -2.004865965629286872 ) ) ;
#4509=AXIS2_PLACEMENT_3D ( 'NONE', #3196, #1058, #1362 ) ;
#4510=TOROIDAL_SURFACE ( 'NONE', #2748, 1.000000000000000000, 0.5000000000000000000 ) ;
#4512=CARTESIAN_POINT ( 'NONE',  ( 190.0000000000000568, 16.03993994372673981, -7.458121719691109004E-14 ) ) ;
#4519=ORIENTED_EDGE ( 'NONE', *, *, #11732, .T. ) ;
#4528=ORIENTED_EDGE ( 'NONE', *, *, #6461, .F. ) ;
#4534=CARTESIAN_POINT ( 'NONE',  ( -64.00000000000002842, 16.03993994372673981, -17.50000000000002487 ) ) ;
#4535=EDGE_CURVE ( 'NONE', #14360, #8201, #5912, .T. ) ;
#4536=AXIS2_PLACEMENT_3D ( 'NONE', #6745, #710, #5553 ) ;
#4540=DIRECTION ( 'NONE',  ( -0.000000000000000000, -0.000000000000000000, 1.000000000000000000 ) ) ;
#4547=CARTESIAN_POINT ( 'NONE',  ( 190.5000000000000568, -178.8058001507315566, 53.19066787724494816 ) ) ;
#4550=AXIS2_PLACEMENT_3D ( 'NONE', #10118, #13648, #2855 ) ;
#4551=DIRECTION ( 'NONE',  ( 0.000000000000000000, -0.000000000000000000, 1.000000000000000000 ) ) ;
#4552=CARTESIAN_POINT ( 'NONE',  ( -76.50000000000001421, 15.53993994372673981, 10.05257423913146475 ) ) ;
#4563=CYLINDRICAL_SURFACE ( 'NONE', #5052, 0.5000000000000004441 ) ;
#4566=ORIENTED_EDGE ( 'NONE', *, *, #15014, .F. ) ;
#4568=CARTESIAN_POINT ( 'NONE',  ( 0.000000000000000000, 0.000000000000000000, 0.000000000000000000 ) ) ;
#4570=CARTESIAN_POINT ( 'NONE',  ( -76.50000000000004263, 17.53993994372673626, 52.49999999999997868 ) ) ;
#4574=CARTESIAN_POINT ( 'NONE',  ( 177.5000000000000853, 15.03993994372673804, 37.07518420361041933 ) ) ;
#4575=VECTOR ( 'NONE', #14907, 1000.000000000000000 ) ;
#4576=AXIS2_PLACEMENT_3D ( 'NONE', #1441, #251, #13210 ) ;
#4578=EDGE_CURVE ( 'NONE', #12077, #13002, #9545, .T. ) ;
#4580=DIRECTION ( 'NONE',  ( -5.518327896226369609E-17, -0.9902680687415712502, -0.1391731009600584990 ) ) ;
#4581=ORIENTED_EDGE ( 'NONE', *, *, #5761, .F. ) ;
#4586=ORIENTED_EDGE ( 'NONE', *, *, #5953, .F. ) ;
#4587=VECTOR ( 'NONE', #13076, 1000.000000000000000 ) ;
#4588=DIRECTION ( 'NONE',  ( 0.000000000000000000, 0.000000000000000000, -1.000000000000000000 ) ) ;
#4590=ORIENTED_EDGE ( 'NONE', *, *, #8098, .F. ) ;
#4596=EDGE_CURVE ( 'NONE', #830, #7696, #8533, .T. ) ;
#4597=ADVANCED_FACE ( 'NONE', ( #13005 ), #9284, .T. ) ;
#4602=DIRECTION ( 'NONE',  ( 0.000000000000000000, 0.000000000000000000, 1.000000000000000000 ) ) ;
#4603=LINE ( 'NONE', #15323, #14124 ) ;
#4608=ORIENTED_EDGE ( 'NONE', *, *, #15503, .F. ) ;
#4613=CARTESIAN_POINT ( 'NONE',  ( -64.00000000000002842, 15.10952649420676686, 25.44255979523916977 ) ) ;
#4618=ORIENTED_EDGE ( 'NONE', *, *, #10848, .F. ) ;
#4620=CIRCLE ( 'NONE', #8921, 0.5000000000000004441 ) ;
#4625=ORIENTED_EDGE ( 'NONE', *, *, #14912, .F. ) ;
#4626=ORIENTED_EDGE ( 'NONE', *, *, #8290, .T. ) ;
#4627=DIRECTION ( 'NONE',  ( -0.000000000000000000, 0.9902680687415711391, 0.1391731009600592484 ) ) ;
#4641=ORIENTED_EDGE ( 'NONE', *, *, #12964, .T. ) ;
#4642=AXIS2_PLACEMENT_3D ( 'NONE', #45, #8370, #12055 ) ;
#4643=VERTEX_POINT ( 'NONE', #10095 ) ;
#4645=AXIS2_PLACEMENT_3D ( 'NONE', #144, #4985, #13420 ) ;
#4647=LINE ( 'NONE', #8302, #4906 ) ;
#4648=DIRECTION ( 'NONE',  ( 0.000000000000000000, -1.000000000000000000, 0.000000000000000000 ) ) ;
#4653=ORIENTED_EDGE ( 'NONE', *, *, #15388, .F. ) ;
#4655=DIRECTION ( 'NONE',  ( -3.965082230804130220E-16, 0.000000000000000000, -1.000000000000000000 ) ) ;
#4666=ORIENTED_EDGE ( 'NONE', *, *, #11197, .T. ) ;
#4671=VERTEX_POINT ( 'NONE', #12373 ) ;
#4673=VECTOR ( 'NONE', #14949, 1000.000000000000000 ) ;
#4676=DIRECTION ( 'NONE',  ( 0.000000000000000000, -4.956352788505162775E-17, 1.000000000000000000 ) ) ;
#4677=FACE_OUTER_BOUND ( 'NONE', #15555, .T. ) ;
#4684=VECTOR ( 'NONE', #9075, 1000.000000000000000 ) ;
#4685=CARTESIAN_POINT ( 'NONE',  ( -63.50000000000002842, 15.53993994372673981, -17.50000000000002487 ) ) ;
#4689=CIRCLE ( 'NONE', #6982, 0.5000000000000004441 ) ;
#4690=ORIENTED_EDGE ( 'NONE', *, *, #1874, .T. ) ;
#4697=DIRECTION ( 'NONE',  ( -5.518327896226369609E-17, 0.9902680687415712502, 0.1391731009600584990 ) ) ;
#4698=DIRECTION ( 'NONE',  ( 0.000000000000000000, 0.9902680687415710281, -0.1391731009600611635 ) ) ;
#4699=AXIS2_PLACEMENT_3D ( 'NONE', #11130, #2756, #1715 ) ;
#4701=TOROIDAL_SURFACE ( 'NONE', #13770, 1.000000000000000000, 0.5000000000000000000 ) ;
#4704=ADVANCED_FACE ( 'NONE', ( #14804 ), #11276, .F. ) ;
#4707=DIRECTION ( 'NONE',  ( 0.000000000000000000, -6.938893903907227145E-17, 1.000000000000000000 ) ) ;
#4712=LINE ( 'NONE', #918, #3611 ) ;
#4715=CARTESIAN_POINT ( 'NONE',  ( 177.5000000000000853, 15.53993994372673626, 52.49999999999997868 ) ) ;
#4722=DIRECTION ( 'NONE',  ( -1.000000000000000000, -0.000000000000000000, -0.000000000000000000 ) ) ;
#4724=CARTESIAN_POINT ( 'NONE',  ( -64.00000000000002842, -178.8058001507315566, -18.19066787724516843 ) ) ;
#4727=CARTESIAN_POINT ( 'NONE',  ( -76.00000000000001421, -179.8058001507315566, -30.31842631998718574 ) ) ;
#4730=EDGE_CURVE ( 'NONE', #9280, #10751, #4476, .T. ) ;
#4738=ORIENTED_EDGE ( 'NONE', *, *, #989, .F. ) ;
#4740=LINE ( 'NONE', #7285, #8054 ) ;
#4742=ORIENTED_EDGE ( 'NONE', *, *, #2088, .F. ) ;
#4743=VECTOR ( 'NONE', #5549, 1000.000000000000000 ) ;
#4744=CARTESIAN_POINT ( 'NONE',  ( -64.00000000000002842, 15.03993994372673804, 37.07518420361041933 ) ) ;
#4748=ORIENTED_EDGE ( 'NONE', *, *, #5403, .F. ) ;
#4759=ORIENTED_EDGE ( 'NONE', *, *, #5973, .F. ) ;
#4763=ORIENTED_EDGE ( 'NONE', *, *, #7953, .T. ) ;
#4765=CARTESIAN_POINT ( 'NONE',  ( 190.5000000000000568, 14.90076684276668040, -2.084916134869001958 ) ) ;
#4766=AXIS2_PLACEMENT_3D ( 'NONE', #10576, #9472, #1010 ) ;
#4767=EDGE_CURVE ( 'NONE', #7175, #14434, #13545, .T. ) ;
#4772=EDGE_CURVE ( 'NONE', #7619, #13426, #2717, .T. ) ;
#4773=DIRECTION ( 'NONE',  ( 1.000000000000000000, 0.000000000000000000, 0.000000000000000000 ) ) ;
#4779=VECTOR ( 'NONE', #14304, 1000.000000000000000 ) ;
#4781=ORIENTED_EDGE ( 'NONE', *, *, #4093, .T. ) ;
#4785=ORIENTED_EDGE ( 'NONE', *, *, #8785, .T. ) ;
#4786=DIRECTION ( 'NONE',  ( -0.000000000000000000, -4.956352788505162775E-17, 1.000000000000000000 ) ) ;
#4791=DIRECTION ( 'NONE',  ( -0.000000000000000000, -1.000000000000000000, -0.000000000000000000 ) ) ;
#4803=FACE_OUTER_BOUND ( 'NONE', #6266, .T. ) ;
#4811=CARTESIAN_POINT ( 'NONE',  ( 178.0000000000000853, -178.8058001507315566, 65.31842631998698323 ) ) ;
#4813=CARTESIAN_POINT ( 'NONE',  ( 177.5000000000000853, 15.10952649420676863, 9.557440204760681013 ) ) ;
#4816=AXIS2_PLACEMENT_3D ( 'NONE', #3568, #8405, #13182 ) ;
#4817=ORIENTED_EDGE ( 'NONE', *, *, #12096, .F. ) ;
#4826=CARTESIAN_POINT ( 'NONE',  ( -76.50000000000001421, -178.8058001507315566, -30.31842631998718574 ) ) ;
#4827=CARTESIAN_POINT ( 'NONE',  ( -63.50000000000002842, 16.03993994372673626, 52.49999999999997868 ) ) ;
#4829=ORIENTED_EDGE ( 'NONE', *, *, #6167, .T. ) ;
#4830=EDGE_CURVE ( 'NONE', #4850, #9446, #3222, .T. ) ;
#4831=FACE_OUTER_BOUND ( 'NONE', #12788, .T. ) ;
#4832=DIRECTION ( 'NONE',  ( 0.000000000000000000, 6.938893903907227145E-17, -1.000000000000000000 ) ) ;
#4841=AXIS2_PLACEMENT_3D ( 'NONE', #8467, #6965, #3401 ) ;
#4843=LINE ( 'NONE', #11791, #10724 ) ;
#4844=FACE_OUTER_BOUND ( 'NONE', #2312, .T. ) ;
#4845=CYLINDRICAL_SURFACE ( 'NONE', #8071, 1.499999999999994449 ) ;
#4850=VERTEX_POINT ( 'NONE', #3297 ) ;
#4853=FACE_OUTER_BOUND ( 'NONE', #14730, .T. ) ;
#4855=TOROIDAL_SURFACE ( 'NONE', #1314, 1.000000000000000000, 0.5000000000000000000 ) ;
#4864=EDGE_CURVE ( 'NONE', #13446, #6990, #8774, .T. ) ;
#4865=DIRECTION ( 'NONE',  ( 1.000000000000000000, 0.000000000000000000, 0.000000000000000000 ) ) ;
#4869=CARTESIAN_POINT ( 'NONE',  ( -63.50000000000002842, -178.9449732516916072, -29.32815825124560760 ) ) ;
#4870=ORIENTED_EDGE ( 'NONE', *, *, #13262, .T. ) ;
#4873=DIRECTION ( 'NONE',  ( -1.000000000000000000, 0.000000000000000000, 0.000000000000000000 ) ) ;
#4876=DIRECTION ( 'NONE',  ( 0.000000000000000000, -0.000000000000000000, 1.000000000000000000 ) ) ;
#4877=DIRECTION ( 'NONE',  ( -0.000000000000000000, 1.000000000000000000, 6.938893903907227145E-17 ) ) ;
#4879=CIRCLE ( 'NONE', #15446, 1.499999999999994449 ) ;
#4881=FACE_OUTER_BOUND ( 'NONE', #5835, .T. ) ;
#4885=DIRECTION ( 'NONE',  ( -1.000000000000000000, -0.000000000000000000, -0.000000000000000000 ) ) ;
#4890=CARTESIAN_POINT ( 'NONE',  ( 177.5000000000000853, -179.8058001507315566, -51.45141194869120227 ) ) ;
#4892=CYLINDRICAL_SURFACE ( 'NONE', #10676, 0.5000000000000004441 ) ;
#4895=ADVANCED_FACE ( 'NONE', ( #11672 ), #833, .T. ) ;
#4898=AXIS2_PLACEMENT_3D ( 'NONE', #9530, #14645, #3763 ) ;
#4902=EDGE_LOOP ( 'NONE', ( #6966, #12151, #8726, #1661 ) ) ;
#4906=VECTOR ( 'NONE', #13083, 1000.000000000000000 ) ;
#4908=ORIENTED_EDGE ( 'NONE', *, *, #13060, .T. ) ;
#4909=LINE ( 'NONE', #9647, #6799 ) ;
#4911=EDGE_CURVE ( 'NONE', #11614, #2480, #426, .T. ) ;
#4923=VECTOR ( 'NONE', #15169, 1000.000000000000000 ) ;
#4932=AXIS2_PLACEMENT_3D ( 'NONE', #10127, #5621, #2943 ) ;
#4937=DIRECTION ( 'NONE',  ( 0.000000000000000000, 0.000000000000000000, 1.000000000000000000 ) ) ;
#4938=DIRECTION ( 'NONE',  ( 3.965082230804130220E-16, 0.000000000000000000, 1.000000000000000000 ) ) ;
#4940=EDGE_CURVE ( 'NONE', #5473, #15212, #2464, .T. ) ;
#4951=CARTESIAN_POINT ( 'NONE',  ( -61.94838851346079167, 15.03993994372673804, 24.94742576086838781 ) ) ;
#4956=CYLINDRICAL_SURFACE ( 'NONE', #3138, 0.5000000000000004441 ) ;
#4958=ADVANCED_FACE ( 'NONE', ( #7969, #5433 ), #10248, .T. ) ;
#4962=ORIENTED_EDGE ( 'NONE', *, *, #537, .T. ) ;
#4963=ORIENTED_EDGE ( 'NONE', *, *, #7499, .T. ) ;
#4971=EDGE_CURVE ( 'NONE', #101, #6346, #13042, .T. ) ;
#4972=VERTEX_POINT ( 'NONE', #3253 ) ;
#4973=ORIENTED_EDGE ( 'NONE', *, *, #5483, .T. ) ;
#4977=CARTESIAN_POINT ( 'NONE',  ( -61.94838851346079167, 15.03993994372673981, -2.575184203610571654 ) ) ;
#4985=DIRECTION ( 'NONE',  ( 0.000000000000000000, -1.000000000000000000, -4.956352788505162775E-17 ) ) ;
#4986=CARTESIAN_POINT ( 'NONE',  ( 190.0000000000000853, 23.05038067821379499, 35.93956260393299829 ) ) ;
#4987=CARTESIAN_POINT ( 'NONE',  ( 177.5000000000000853, 15.53993994372673981, -17.50000000000002487 ) ) ;
#4989=CIRCLE ( 'NONE', #12290, 0.5000000000000001110 ) ;
#4991=ADVANCED_FACE ( 'NONE', ( #10678 ), #2064, .T. ) ;
#4995=VERTEX_POINT ( 'NONE', #12313 ) ;
#5004=ORIENTED_EDGE ( 'NONE', *, *, #15572, .F. ) ;
#5005=DIRECTION ( 'NONE',  ( 0.000000000000000000, 0.000000000000000000, 1.000000000000000000 ) ) ;
#5006=DIRECTION ( 'NONE',  ( 1.000000000000000000, -0.000000000000000000, -0.000000000000000000 ) ) ;
#5009=AXIS2_PLACEMENT_3D ( 'NONE', #13508, #2872, #14845 ) ;
#5012=VECTOR ( 'NONE', #648, 1000.000000000000000 ) ;
#5013=CARTESIAN_POINT ( 'NONE',  ( -64.00000000000002842, 15.53993994372673981, 9.617930870223348805 ) ) ;
#5019=DIRECTION ( 'NONE',  ( -1.000000000000000000, 0.000000000000000000, 0.000000000000000000 ) ) ;
#5020=VERTEX_POINT ( 'NONE', #11064 ) ;
#5025=AXIS2_PLACEMENT_3D ( 'NONE', #14116, #11761, #5756 ) ;
#5027=DIRECTION ( 'NONE',  ( -0.000000000000000000, -4.956352788505162775E-17, 1.000000000000000000 ) ) ;
#5038=EDGE_CURVE ( 'NONE', #3389, #13605, #1263, .T. ) ;
#5039=ORIENTED_EDGE ( 'NONE', *, *, #3750, .F. ) ;
#5041=DIRECTION ( 'NONE',  ( -0.000000000000000000, 1.000000000000000000, 6.938893903907227145E-17 ) ) ;
#5045=CARTESIAN_POINT ( 'NONE',  ( -76.00000000000004263, 15.53993994372673804, 38.07518420361041933 ) ) ;
#5052=AXIS2_PLACEMENT_3D ( 'NONE', #923, #5750, #8223 ) ;
#5053=AXIS2_PLACEMENT_3D ( 'NONE', #5417, #9055, #13854 ) ;
#5058=ORIENTED_EDGE ( 'NONE', *, *, #9272, .T. ) ;
#5062=DIRECTION ( 'NONE',  ( -1.000000000000000000, 0.000000000000000000, 0.000000000000000000 ) ) ;
#5064=AXIS2_PLACEMENT_3D ( 'NONE', #1419, #4832, #6252 ) ;
#5067=DIRECTION ( 'NONE',  ( 1.000000000000000000, 0.000000000000000000, 0.000000000000000000 ) ) ;
#5073=ORIENTED_EDGE ( 'NONE', *, *, #6450, .F. ) ;
#5076=ORIENTED_EDGE ( 'NONE', *, *, #1897, .T. ) ;
#5077=VERTEX_POINT ( 'NONE', #7290 ) ;
#5078=AXIS2_PLACEMENT_3D ( 'NONE', #15459, #4655, #5850 ) ;
#5083=ADVANCED_FACE ( 'NONE', ( #3950 ), #14446, .T. ) ;
#5084=EDGE_CURVE ( 'NONE', #14585, #3344, #5657, .T. ) ;
#5087=AXIS2_PLACEMENT_3D ( 'NONE', #1730, #1808, #7754 ) ;
#5089=DIRECTION ( 'NONE',  ( 0.000000000000000000, 0.9902680687415711391, 0.1391731009600593039 ) ) ;
#5092=CARTESIAN_POINT ( 'NONE',  ( -76.00000000000004263, 14.90076684276667862, 37.08491613486884830 ) ) ;
#5096=ORIENTED_EDGE ( 'NONE', *, *, #6908, .F. ) ;
#5098=CIRCLE ( 'NONE', #2577, 1.000000000000000888 ) ;
#5101=VERTEX_POINT ( 'NONE', #6180 ) ;
#5102=CIRCLE ( 'NONE', #3845, 0.5000000000000004441 ) ;
#5106=DIRECTION ( 'NONE',  ( 1.000000000000000000, 0.000000000000000000, 0.000000000000000000 ) ) ;
#5107=AXIS2_PLACEMENT_3D ( 'NONE', #13496, #6577, #11379 ) ;
#5112=DIRECTION ( 'NONE',  ( 0.000000000000000000, -1.000000000000000000, -4.956352788505162775E-17 ) ) ;
#5114=CARTESIAN_POINT ( 'NONE',  ( 177.5000000000000853, -179.8058001507315566, 65.31842631998698323 ) ) ;
#5115=ADVANCED_FACE ( 'NONE', ( #75 ), #6333, .F. ) ;
#5118=CARTESIAN_POINT ( 'NONE',  ( 190.0000000000000568, -179.8058001507315566, -17.50000000000002487 ) ) ;
#5120=DIRECTION ( 'NONE',  ( 0.000000000000000000, 1.000000000000000000, 6.938893903907227145E-17 ) ) ;
#5123=FACE_OUTER_BOUND ( 'NONE', #10624, .T. ) ;
#5124=AXIS2_PLACEMENT_3D ( 'NONE', #10270, #4492, #619 ) ;
#5128=DIRECTION ( 'NONE',  ( 0.000000000000000000, 0.000000000000000000, 1.000000000000000000 ) ) ;
#5130=ADVANCED_FACE ( 'NONE', ( #4831 ), #10168, .T. ) ;
#5132=ORIENTED_EDGE ( 'NONE', *, *, #12628, .F. ) ;
#5139=ORIENTED_EDGE ( 'NONE', *, *, #12205, .T. ) ;
#5143=CARTESIAN_POINT ( 'NONE',  ( -61.94838851346079167, -181.3058001507315566, 84.88378295107885663 ) ) ;
#5148=DIRECTION ( 'NONE',  ( 0.000000000000000000, 0.000000000000000000, -1.000000000000000000 ) ) ;
#5152=EDGE_CURVE ( 'NONE', #4850, #5311, #6251, .T. ) ;
#5153=DIRECTION ( 'NONE',  ( 0.000000000000000000, 0.000000000000000000, 1.000000000000000000 ) ) ;
#5155=ORIENTED_EDGE ( 'NONE', *, *, #7500, .F. ) ;
#5160=DIRECTION ( 'NONE',  ( -1.000000000000000000, 0.000000000000000000, 0.000000000000000000 ) ) ;
#5170=DIRECTION ( 'NONE',  ( 0.000000000000000000, -1.000000000000000000, 0.000000000000000000 ) ) ;
#5177=EDGE_LOOP ( 'NONE', ( #7110, #11271, #4443, #10831 ) ) ;
#5180=PLANE ( 'NONE',  #1606 ) ;
#5181=CARTESIAN_POINT ( 'NONE',  ( -70.00000000000000000, -181.3058001507315566, 74.95141194869098911 ) ) ;
#5184=DIRECTION ( 'NONE',  ( 3.965082230804130220E-16, 4.956352788505162775E-17, -1.000000000000000000 ) ) ;
#5186=ADVANCED_FACE ( 'NONE', ( #15059, #10267 ), #5374, .F. ) ;
#5187=EDGE_CURVE ( 'NONE', #6271, #2702, #10927, .T. ) ;
#5189=DIRECTION ( 'NONE',  ( -0.000000000000000000, -0.9902680687415712502, -0.1391731009600586100 ) ) ;
#5191=EDGE_LOOP ( 'NONE', ( #896, #4973, #15325, #3038 ) ) ;
#5202=ORIENTED_EDGE ( 'NONE', *, *, #534, .T. ) ;
#5203=ADVANCED_FACE ( 'NONE', ( #3087 ), #9092, .T. ) ;
#5218=ADVANCED_FACE ( 'NONE', ( #10346 ), #10117, .F. ) ;
#5219=CARTESIAN_POINT ( 'NONE',  ( -64.00000000000002842, -178.8058001507315566, 52.69066787724494816 ) ) ;
#5220=VERTEX_POINT ( 'NONE', #12700 ) ;
#5227=DIRECTION ( 'NONE',  ( -1.000000000000000000, -2.751328491981765035E-32, 3.965082230804130220E-16 ) ) ;
#5228=VERTEX_POINT ( 'NONE', #6493 ) ;
#5235=CARTESIAN_POINT ( 'NONE',  ( -76.00000000000004263, -179.8058001507315566, 52.19066787724494816 ) ) ;
#5239=EDGE_LOOP ( 'NONE', ( #5753, #9600, #290, #3891 ) ) ;
#5240=CYLINDRICAL_SURFACE ( 'NONE', #5078, 0.5000000000000004441 ) ;
#5249=CARTESIAN_POINT ( 'NONE',  ( -61.94838851346079167, 15.53993994372673981, -2.500000000000070610 ) ) ;
#5250=DIRECTION ( 'NONE',  ( 0.000000000000000000, -1.000000000000000000, -4.956352788505162775E-17 ) ) ;
#5253=AXIS2_PLACEMENT_3D ( 'NONE', #7960, #12748, #8908 ) ;
#5265=ORIENTED_EDGE ( 'NONE', *, *, #1602, .F. ) ;
#5266=VERTEX_POINT ( 'NONE', #9012 ) ;
#5268=CARTESIAN_POINT ( 'NONE',  ( 190.0000000000000568, 16.03993994372673981, 24.94742576086838781 ) ) ;
#5273=EDGE_CURVE ( 'NONE', #10340, #8004, #6929, .T. ) ;
#5275=ADVANCED_FACE ( 'NONE', ( #4333 ), #2934, .T. ) ;
#5276=TOROIDAL_SURFACE ( 'NONE', #7309, 1.000000000000000000, 0.5000000000000000000 ) ;
#5278=AXIS2_PLACEMENT_3D ( 'NONE', #10614, #15404, #14381 ) ;
#5281=DIRECTION ( 'NONE',  ( 1.000000000000000000, 0.000000000000000000, 0.000000000000000000 ) ) ;
#5282=CIRCLE ( 'NONE', #3774, 0.5000000000000004441 ) ;
#5288=ORIENTED_EDGE ( 'NONE', *, *, #11449, .T. ) ;
#5293=FACE_OUTER_BOUND ( 'NONE', #12041, .T. ) ;
#5296=ORIENTED_EDGE ( 'NONE', *, *, #6614, .F. ) ;
#5298=ORIENTED_EDGE ( 'NONE', *, *, #8566, .F. ) ;
#5305=EDGE_LOOP ( 'NONE', ( #3629, #13158, #9901, #5139 ) ) ;
#5309=VECTOR ( 'NONE', #10690, 1000.000000000000000 ) ;
#5311=VERTEX_POINT ( 'NONE', #375 ) ;
#5312=AXIS2_PLACEMENT_3D ( 'NONE', #13935, #4451, #9135 ) ;
#5314=CARTESIAN_POINT ( 'NONE',  ( 177.5000000000000853, -181.3058001507315566, 84.88378295107885663 ) ) ;
#5324=DIRECTION ( 'NONE',  ( 3.965082230804130220E-16, 1.090924371466202084E-47, 1.000000000000000000 ) ) ;
#5325=ORIENTED_EDGE ( 'NONE', *, *, #8305, .T. ) ;
#5330=AXIS2_PLACEMENT_3D ( 'NONE', #11219, #13644, #7512 ) ;
#5335=CARTESIAN_POINT ( 'NONE',  ( 190.5000000000000853, -178.9449732516916072, 64.32815825124538378 ) ) ;
#5343=AXIS2_PLACEMENT_3D ( 'NONE', #8394, #13171, #8162 ) ;
#5346=CARTESIAN_POINT ( 'NONE',  ( -76.50000000000001421, -179.2362136002515172, -18.26098611522645498 ) ) ;
#5347=ADVANCED_FACE ( 'NONE', ( #10501 ), #8203, .T. ) ;
#5349=ORIENTED_EDGE ( 'NONE', *, *, #1926, .F. ) ;
#5355=STYLED_ITEM ( 'NONE', ( #4051 ), #10819 ) ;
#5363=DIRECTION ( 'NONE',  ( 1.000000000000000000, 2.751328491981765035E-32, -3.965082230804130220E-16 ) ) ;
#5365=ORIENTED_EDGE ( 'NONE', *, *, #13754, .T. ) ;
#5369=VERTEX_POINT ( 'NONE', #15524 ) ;
#5374=PLANE ( 'NONE',  #8946 ) ;
#5386=CARTESIAN_POINT ( 'NONE',  ( -64.00000000000002842, -179.3058001507315566, -51.45141194869120227 ) ) ;
#5390=ORIENTED_EDGE ( 'NONE', *, *, #6228, .F. ) ;
#5391=ORIENTED_EDGE ( 'NONE', *, *, #1187, .T. ) ;
#5394=ORIENTED_EDGE ( 'NONE', *, *, #1764, .T. ) ;
#5400=CARTESIAN_POINT ( 'NONE',  ( 184.0000000000000568, 15.53993994372673626, 48.99999999999997158 ) ) ;
#5402=VECTOR ( 'NONE', #5027, 1000.000000000000000 ) ;
#5403=EDGE_CURVE ( 'NONE', #14746, #14786, #4647, .T. ) ;
#5404=CARTESIAN_POINT ( 'NONE',  ( -76.00000000000007105, -178.8058001507315566, 65.31842631998698323 ) ) ;
#5405=ORIENTED_EDGE ( 'NONE', *, *, #1989, .T. ) ;
#5406=DIRECTION ( 'NONE',  ( 0.000000000000000000, 0.000000000000000000, 1.000000000000000000 ) ) ;
#5409=DIRECTION ( 'NONE',  ( 3.965082230804130220E-16, 1.090924371466202084E-47, 1.000000000000000000 ) ) ;
#5413=AXIS2_PLACEMENT_3D ( 'NONE', #13972, #3158, #11221 ) ;
#5415=DIRECTION ( 'NONE',  ( -0.000000000000000000, -0.9902680687415713612, 0.1391731009600582492 ) ) ;
#5417=CARTESIAN_POINT ( 'NONE',  ( 190.0000000000000568, 15.03993994372673981, -3.075184203610571654 ) ) ;
#5418=CIRCLE ( 'NONE', #10468, 0.5000000000000004441 ) ;
#5423=DIRECTION ( 'NONE',  ( 0.000000000000000000, 0.000000000000000000, -1.000000000000000000 ) ) ;
#5429=AXIS2_PLACEMENT_3D ( 'NONE', #3039, #12804, #5406 ) ;
#5433=FACE_OUTER_BOUND ( 'NONE', #6447, .T. ) ;
#5435=CARTESIAN_POINT ( 'NONE',  ( 178.0000000000000853, -179.8058001507315566, 52.19066787724494816 ) ) ;
#5438=MANIFOLD_SOLID_BREP ( 'Cut-Extrude3', #11920 ) ;
#5440=EDGE_CURVE ( 'NONE', #13575, #11344, #10452, .T. ) ;
#5441=CARTESIAN_POINT ( 'NONE',  ( 190.0000000000000853, -179.3058001507316419, 52.76585208085545986 ) ) ;
#5444=AXIS2_PLACEMENT_3D ( 'NONE', #322, #5160, #161 ) ;
#5445=CARTESIAN_POINT ( 'NONE',  ( 177.5000000000000853, -179.8058001507315566, 52.19066787724494816 ) ) ;
#5450=CARTESIAN_POINT ( 'NONE',  ( 190.0000000000000568, 15.53993994372673981, 10.05257423913146475 ) ) ;
#5454=CARTESIAN_POINT ( 'NONE',  ( -61.94838851346079167, -179.3058001507315566, -51.45141194869120227 ) ) ;
#5460=EDGE_CURVE ( 'NONE', #4643, #3604, #3624, .T. ) ;
#5462=ORIENTED_EDGE ( 'NONE', *, *, #10682, .F. ) ;
#5464=ADVANCED_FACE ( 'NONE', ( #54 ), #4892, .T. ) ;
#5472=ORIENTED_EDGE ( 'NONE', *, *, #12782, .F. ) ;
#5473=VERTEX_POINT ( 'NONE', #11045 ) ;
#5475=DIRECTION ( 'NONE',  ( 0.000000000000000000, -1.000000000000000000, -6.938893903907227145E-17 ) ) ;
#5476=ORIENTED_EDGE ( 'NONE', *, *, #15398, .T. ) ;
#5483=EDGE_CURVE ( 'NONE', #3488, #7175, #3866, .T. ) ;
#5485=EDGE_LOOP ( 'NONE', ( #14630, #10433 ) ) ;
#5489=ORIENTED_EDGE ( 'NONE', *, *, #11728, .F. ) ;
#5492=EDGE_LOOP ( 'NONE', ( #6776, #541, #4618, #11953 ) ) ;
#5497=CIRCLE ( 'NONE', #12565, 0.5000000000000001110 ) ;
#5499=ORIENTED_EDGE ( 'NONE', *, *, #14232, .T. ) ;
#5501=DIRECTION ( 'NONE',  ( 0.000000000000000000, 0.000000000000000000, 1.000000000000000000 ) ) ;
#5518=CARTESIAN_POINT ( 'NONE',  ( 190.0000000000000568, 15.53993994372673804, 25.38206912977649310 ) ) ;
#5521=DIRECTION ( 'NONE',  ( 0.000000000000000000, 1.000000000000000000, 0.000000000000000000 ) ) ;
#5522=CIRCLE ( 'NONE', #13827, 0.5000000000000001110 ) ;
#5524=EDGE_CURVE ( 'NONE', #4850, #2407, #14688, .T. ) ;
#5529=DIRECTION ( 'NONE',  ( 1.000000000000000000, 0.000000000000000000, 0.000000000000000000 ) ) ;
#5532=DIRECTION ( 'NONE',  ( 0.000000000000000000, 0.000000000000000000, -1.000000000000000000 ) ) ;
#5534=VECTOR ( 'NONE', #13416, 1000.000000000000000 ) ;
#5540=CIRCLE ( 'NONE', #460, 1.500000000000001332 ) ;
#5545=CIRCLE ( 'NONE', #7780, 0.5000000000000004441 ) ;
#5549=DIRECTION ( 'NONE',  ( -0.000000000000000000, -0.000000000000000000, 1.000000000000000000 ) ) ;
#5553=DIRECTION ( 'NONE',  ( 0.000000000000000000, -3.469446951953611033E-15, 1.000000000000000000 ) ) ;
#5555=CYLINDRICAL_SURFACE ( 'NONE', #994, 0.5000000000000004441 ) ;
#5556=DIRECTION ( 'NONE',  ( -0.000000000000000000, 1.000000000000000000, 6.938893903907227145E-17 ) ) ;
#5557=CIRCLE ( 'NONE', #14828, 0.5000000000000004441 ) ;
#5558=DIRECTION ( 'NONE',  ( 0.000000000000000000, 0.000000000000000000, -1.000000000000000000 ) ) ;
#5559=AXIS2_PLACEMENT_3D ( 'NONE', #11316, #15010, #4200 ) ;
#5563=CARTESIAN_POINT ( 'NONE',  ( 178.0000000000000853, -179.3058001507315566, -17.19066787724516843 ) ) ;
#5564=AXIS2_PLACEMENT_3D ( 'NONE', #2952, #12486, #1677 ) ;
#5576=DIRECTION ( 'NONE',  ( 1.000000000000000000, -2.751328491981765035E-32, 3.965082230804130220E-16 ) ) ;
#5577=CIRCLE ( 'NONE', #14376, 0.5000000000000004441 ) ;
#5579=VECTOR ( 'NONE', #8749, 1000.000000000000000 ) ;
#5581=DIRECTION ( 'NONE',  ( 1.000000000000000000, -0.000000000000000000, -0.000000000000000000 ) ) ;
#5583=FACE_OUTER_BOUND ( 'NONE', #3116, .T. ) ;
#5587=ORIENTED_EDGE ( 'NONE', *, *, #2062, .T. ) ;
#5591=ORIENTED_EDGE ( 'NONE', *, *, #12594, .F. ) ;
#5600=CARTESIAN_POINT ( 'NONE',  ( -76.50000000000004263, -178.6666270497714777, 53.18093594598651919 ) ) ;
#5608=CARTESIAN_POINT ( 'NONE',  ( 190.0000000000000568, -179.8058001507315566, -51.45141194869120937 ) ) ;
#5609=CIRCLE ( 'NONE', #10390, 0.5000000000000004441 ) ;
#5610=ORIENTED_EDGE ( 'NONE', *, *, #731, .F. ) ;
#5613=CARTESIAN_POINT ( 'NONE',  ( 0.000000000000000000, 15.03993994372673804, 38.07518420361041933 ) ) ;
#5614=ORIENTED_EDGE ( 'NONE', *, *, #1929, .T. ) ;
#5620=AXIS2_PLACEMENT_3D ( 'NONE', #4338, #12777, #9249 ) ;
#5621=DIRECTION ( 'NONE',  ( 0.000000000000000000, 1.000000000000000000, 6.938893903907227145E-17 ) ) ;
#5625=ORIENTED_EDGE ( 'NONE', *, *, #921, .F. ) ;
#5630=CYLINDRICAL_SURFACE ( 'NONE', #9086, 0.5000000000000004441 ) ;
#5633=CARTESIAN_POINT ( 'NONE',  ( 184.0000000000000568, 17.53993994372673626, 45.99999999999998579 ) ) ;
#5637=ORIENTED_EDGE ( 'NONE', *, *, #10664, .T. ) ;
#5638=CARTESIAN_POINT ( 'NONE',  ( -76.50000000000001421, 15.03993994372673981, -3.075184203610571654 ) ) ;
#5652=EDGE_LOOP ( 'NONE', ( #4581, #7047, #1555, #7393 ) ) ;
#5653=LINE ( 'NONE', #658, #8397 ) ;
#5657=CIRCLE ( 'NONE', #1329, 0.5000000000000001110 ) ;
#5675=DIRECTION ( 'NONE',  ( 0.000000000000000000, 0.000000000000000000, 1.000000000000000000 ) ) ;
#5677=CARTESIAN_POINT ( 'NONE',  ( -76.50000000000001421, 16.03993994372673981, -3.075184203610571654 ) ) ;
#5679=CARTESIAN_POINT ( 'NONE',  ( 178.0000000000000853, 16.03993994372673981, 10.05257423913146475 ) ) ;
#5680=ORIENTED_EDGE ( 'NONE', *, *, #245, .F. ) ;
#5681=DIRECTION ( 'NONE',  ( 1.000000000000000000, 0.000000000000000000, 0.000000000000000000 ) ) ;
#5682=ORIENTED_EDGE ( 'NONE', *, *, #12839, .F. ) ;
#5692=ORIENTED_EDGE ( 'NONE', *, *, #657, .T. ) ;
#5695=EDGE_LOOP ( 'NONE', ( #4498, #6502, #11540, #5390 ) ) ;
#5696=CARTESIAN_POINT ( 'NONE',  ( 178.0000000000000853, 16.03993994372673981, -3.075184203610571654 ) ) ;
#5697=VECTOR ( 'NONE', #2463, 1000.000000000000114 ) ;
#5698=DIRECTION ( 'NONE',  ( 0.000000000000000000, -1.000000000000000000, -4.956352788505162775E-17 ) ) ;
#5708=DIRECTION ( 'NONE',  ( 0.000000000000000000, 0.000000000000000000, -1.000000000000000000 ) ) ;
#5710=CIRCLE ( 'NONE', #140, 0.5000000000000004441 ) ;
#5712=FACE_OUTER_BOUND ( 'NONE', #11993, .T. ) ;
#5714=DIRECTION ( 'NONE',  ( 0.000000000000000000, 1.000000000000000000, 0.000000000000000000 ) ) ;
#5715=ADVANCED_FACE ( 'NONE', ( #14098 ), #15431, .T. ) ;
#5716=DIRECTION ( 'NONE',  ( 1.000000000000000000, -2.751328491981765035E-32, 3.965082230804130220E-16 ) ) ;
#5723=DIRECTION ( 'NONE',  ( 0.000000000000000000, 1.734723475976805517E-15, 1.000000000000000000 ) ) ;
#5728=LINE ( 'NONE', #10541, #4088 ) ;
#5730=AXIS2_PLACEMENT_3D ( 'NONE', #14892, #14739, #12453 ) ;
#5731=ORIENTED_EDGE ( 'NONE', *, *, #1967, .F. ) ;
#5732=DIRECTION ( 'NONE',  ( -1.000000000000000000, 0.000000000000000000, 0.000000000000000000 ) ) ;
#5735=CARTESIAN_POINT ( 'NONE',  ( -76.00000000000001421, -178.8058001507315566, 52.19066787724494816 ) ) ;
#5738=ORIENTED_EDGE ( 'NONE', *, *, #8613, .F. ) ;
#5748=LINE ( 'NONE', #1948, #14215 ) ;
#5750=DIRECTION ( 'NONE',  ( 3.965082230804130220E-16, 4.956352788505162775E-17, -1.000000000000000000 ) ) ;
#5751=FACE_OUTER_BOUND ( 'NONE', #9926, .T. ) ;
#5753=ORIENTED_EDGE ( 'NONE', *, *, #7218, .T. ) ;
#5755=ORIENTED_EDGE ( 'NONE', *, *, #6228, .T. ) ;
#5756=DIRECTION ( 'NONE',  ( 0.000000000000000000, 0.000000000000000000, 1.000000000000000000 ) ) ;
#5757=EDGE_LOOP ( 'NONE', ( #4339, #6154, #6668, #2379 ) ) ;
#5758=EDGE_CURVE ( 'NONE', #9239, #7288, #1590, .T. ) ;
#5761=EDGE_CURVE ( 'NONE', #138, #6739, #3452, .T. ) ;
#5764=CIRCLE ( 'NONE', #11067, 1.000000000000000444 ) ;
#5768=CARTESIAN_POINT ( 'NONE',  ( 190.0000000000000568, -178.8753867012115961, -29.82329228561640022 ) ) ;
#5770=DIRECTION ( 'NONE',  ( -0.000000000000000000, 0.9902680687415702510, -0.1391731009600660485 ) ) ;
#5774=DIRECTION ( 'NONE',  ( 0.000000000000000000, -1.000000000000000000, -6.938893903907227145E-17 ) ) ;
#5777=VERTEX_POINT ( 'NONE', #15274 ) ;
#5781=AXIS2_PLACEMENT_3D ( 'NONE', #14132, #12711, #2056 ) ;
#5782=EDGE_LOOP ( 'NONE', ( #5680, #7233, #14621, #31 ) ) ;
#5783=DIRECTION ( 'NONE',  ( -5.518327896226364679E-17, -0.9902680687415713612, 0.1391731009600582492 ) ) ;
#5784=VERTEX_POINT ( 'NONE', #11901 ) ;
#5787=CYLINDRICAL_SURFACE ( 'NONE', #484, 0.5000000000000004441 ) ;
#5788=DIRECTION ( 'NONE',  ( 0.000000000000000000, -0.9902680687415713612, 0.1391731009600582492 ) ) ;
#5790=EDGE_LOOP ( 'NONE', ( #9951, #1283 ) ) ;
#5796=AXIS2_PLACEMENT_3D ( 'NONE', #15008, #14062, #5708 ) ;
#5797=AXIS2_PLACEMENT_3D ( 'NONE', #323, #4126, #11398 ) ;
#5798=DIRECTION ( 'NONE',  ( -1.000000000000000000, 0.000000000000000000, 0.000000000000000000 ) ) ;
#5802=ORIENTED_EDGE ( 'NONE', *, *, #14988, .F. ) ;
#5810=DIRECTION ( 'NONE',  ( 0.000000000000000000, -0.1391731009600641333, -0.9902680687415704730 ) ) ;
#5811=DIRECTION ( 'NONE',  ( -3.965082230804130220E-16, 1.090924371466202084E-47, 1.000000000000000000 ) ) ;
#5813=ORIENTED_EDGE ( 'NONE', *, *, #5985, .F. ) ;
#5814=ORIENTED_EDGE ( 'NONE', *, *, #11312, .F. ) ;
#5815=AXIS2_PLACEMENT_3D ( 'NONE', #1885, #12701, #14120 ) ;
#5816=DIRECTION ( 'NONE',  ( 1.000000000000000000, 0.000000000000000000, 0.000000000000000000 ) ) ;
#5827=DIRECTION ( 'NONE',  ( 0.000000000000000000, -4.956352788505162775E-17, 1.000000000000000000 ) ) ;
#5830=CARTESIAN_POINT ( 'NONE',  ( -76.50000000000001421, -179.3058001507315566, 84.88378295107887084 ) ) ;
#5832=CARTESIAN_POINT ( 'NONE',  ( 177.5000000000000853, -179.8058001507315566, -17.19066787724516843 ) ) ;
#5833=ORIENTED_EDGE ( 'NONE', *, *, #10682, .T. ) ;
#5835=EDGE_LOOP ( 'NONE', ( #10237, #1262, #1707, #15397 ) ) ;
#5838=ORIENTED_EDGE ( 'NONE', *, *, #14295, .F. ) ;
#5840=CARTESIAN_POINT ( 'NONE',  ( -63.50000000000002842, -178.8058001507315566, -30.31842631998718574 ) ) ;
#5841=VECTOR ( 'NONE', #7494, 1000.000000000000000 ) ;
#5844=VERTEX_POINT ( 'NONE', #3374 ) ;
#5845=EDGE_LOOP ( 'NONE', ( #5349, #818, #13666, #14377 ) ) ;
#5850=DIRECTION ( 'NONE',  ( -1.000000000000000000, 0.000000000000000000, 0.000000000000000000 ) ) ;
#5852=CARTESIAN_POINT ( 'NONE',  ( -64.00000000000002842, -178.8753867012115961, 64.82329228561619061 ) ) ;
#5853=AXIS2_PLACEMENT_3D ( 'NONE', #2687, #1724, #6560 ) ;
#5865=AXIS2_PLACEMENT_3D ( 'NONE', #9970, #14757, #3953 ) ;
#5867=VERTEX_POINT ( 'NONE', #7255 ) ;
#5868=ADVANCED_FACE ( 'NONE', ( #13222 ), #10717, .T. ) ;
#5880=DIRECTION ( 'NONE',  ( 1.000000000000000000, 2.751328491981765035E-32, -3.965082230804130220E-16 ) ) ;
#5882=PLANE ( 'NONE',  #4509 ) ;
#5883=EDGE_CURVE ( 'NONE', #6990, #5844, #10191, .T. ) ;
#5887=DIRECTION ( 'NONE',  ( -1.000000000000000000, 0.000000000000000000, 0.000000000000000000 ) ) ;
#5891=CYLINDRICAL_SURFACE ( 'NONE', #15614, 0.5000000000000004441 ) ;
#5894=ORIENTED_EDGE ( 'NONE', *, *, #8190, .T. ) ;
#5897=DIRECTION ( 'NONE',  ( 0.000000000000000000, -1.000000000000000000, -4.956352788505160310E-17 ) ) ;
#5898=DIRECTION ( 'NONE',  ( 0.000000000000000000, -0.1391731009600586100, 0.9902680687415712502 ) ) ;
#5905=DIRECTION ( 'NONE',  ( 0.000000000000000000, -0.9902680687415702510, -0.1391731009600660485 ) ) ;
#5906=LINE ( 'NONE', #14490, #10702 ) ;
#5911=VERTEX_POINT ( 'NONE', #13300 ) ;
#5912=LINE ( 'NONE', #4570, #15331 ) ;
#5913=CARTESIAN_POINT ( 'NONE',  ( 184.0000000000000568, -201.3058001507315566, 77.95141194869098911 ) ) ;
#5920=ORIENTED_EDGE ( 'NONE', *, *, #11845, .T. ) ;
#5923=DIRECTION ( 'NONE',  ( 1.000000000000000000, 0.000000000000000000, 0.000000000000000000 ) ) ;
#5930=ORIENTED_EDGE ( 'NONE', *, *, #4730, .F. ) ;
#5933=ADVANCED_FACE ( 'NONE', ( #7178 ), #6216, .F. ) ;
#5934=DIRECTION ( 'NONE',  ( -0.000000000000000000, -6.938893903907227145E-17, 1.000000000000000000 ) ) ;
#5935=EDGE_CURVE ( 'NONE', #5777, #1807, #14451, .T. ) ;
#5936=CIRCLE ( 'NONE', #6200, 0.5000000000000004441 ) ;
#5944=CARTESIAN_POINT ( 'NONE',  ( -64.00000000000002842, 16.03993994372673981, 7.553451883674125344E-16 ) ) ;
#5945=DIRECTION ( 'NONE',  ( 1.000000000000000000, 0.000000000000000000, 0.000000000000000000 ) ) ;
#5953=EDGE_CURVE ( 'NONE', #2480, #2355, #14328, .T. ) ;
#5955=CARTESIAN_POINT ( 'NONE',  ( -64.00000000000002842, -179.3058001507315566, -17.19066787724516843 ) ) ;
#5956=ADVANCED_FACE ( 'NONE', ( #7332 ), #6064, .T. ) ;
#5957=AXIS2_PLACEMENT_3D ( 'NONE', #1758, #6597, #3108 ) ;
#5960=ORIENTED_EDGE ( 'NONE', *, *, #13956, .T. ) ;
#5966=LINE ( 'NONE', #10706, #12228 ) ;
#5973=EDGE_CURVE ( 'NONE', #720, #13191, #585, .T. ) ;
#5975=ORIENTED_EDGE ( 'NONE', *, *, #3442, .F. ) ;
#5976=DIRECTION ( 'NONE',  ( 0.000000000000000000, 0.000000000000000000, 1.000000000000000000 ) ) ;
#5977=PLANE ( 'NONE',  #15106 ) ;
#5979=DIRECTION ( 'NONE',  ( 0.000000000000000000, 0.9902680687415713612, -0.1391731009600582492 ) ) ;
#5983=CARTESIAN_POINT ( 'NONE',  ( -76.00000000000001421, 15.03993994372673981, -2.575184203610571654 ) ) ;
#5985=EDGE_CURVE ( 'NONE', #8328, #427, #3886, .T. ) ;
#5989=DIRECTION ( 'NONE',  ( 1.000000000000000000, 2.751328491981765035E-32, -3.965082230804130220E-16 ) ) ;
#5990=VERTEX_POINT ( 'NONE', #15587 ) ;
#5991=EDGE_CURVE ( 'NONE', #652, #12666, #11413, .T. ) ;
#5998=CARTESIAN_POINT ( 'NONE',  ( -76.00000000000001421, -179.8058001507315566, -17.50000000000002487 ) ) ;
#6003=EDGE_LOOP ( 'NONE', ( #12271, #13908 ) ) ;
#6007=ORIENTED_EDGE ( 'NONE', *, *, #2378, .T. ) ;
#6015=DIRECTION ( 'NONE',  ( -1.000000000000000000, 0.000000000000000000, 0.000000000000000000 ) ) ;
#6016=CYLINDRICAL_SURFACE ( 'NONE', #10103, 0.4999999999999996114 ) ;
#6019=EDGE_CURVE ( 'NONE', #8345, #652, #11702, .T. ) ;
#6021=VECTOR ( 'NONE', #2298, 1000.000000000000114 ) ;
#6027=TOROIDAL_SURFACE ( 'NONE', #4240, 1.000000000000000000, 0.5000000000000000000 ) ;
#6028=EDGE_CURVE ( 'NONE', #235, #6953, #9052, .T. ) ;
#6038=AXIS2_PLACEMENT_3D ( 'NONE', #13591, #14773, #14698 ) ;
#6041=EDGE_LOOP ( 'NONE', ( #14074, #4908, #13529, #351 ) ) ;
#6045=ORIENTED_EDGE ( 'NONE', *, *, #1702, .F. ) ;
#6046=FACE_OUTER_BOUND ( 'NONE', #4091, .T. ) ;
#6047=CARTESIAN_POINT ( 'NONE',  ( -76.50000000000004263, -179.3753867012116530, 64.38864891670806401 ) ) ;
#6049=EDGE_CURVE ( 'NONE', #6990, #12750, #10155, .T. ) ;
#6053=ADVANCED_FACE ( 'NONE', ( #2896 ), #5180, .T. ) ;
#6059=ORIENTED_EDGE ( 'NONE', *, *, #9191, .T. ) ;
#6064=PLANE ( 'NONE',  #7430 ) ;
#6066=CARTESIAN_POINT ( 'NONE',  ( -70.00000000000000000, -179.3058001507315566, 76.45141194869098911 ) ) ;
#6074=DIRECTION ( 'NONE',  ( 3.965082230804130220E-16, -0.000000000000000000, -1.000000000000000000 ) ) ;
#6077=VERTEX_POINT ( 'NONE', #7719 ) ;
#6079=VERTEX_POINT ( 'NONE', #6530 ) ;
#6084=CARTESIAN_POINT ( 'NONE',  ( 190.5000000000000568, -179.8058001507315566, 84.88378295107887084 ) ) ;
#6086=DIRECTION ( 'NONE',  ( 1.000000000000000000, 0.000000000000000000, 0.000000000000000000 ) ) ;
#6087=CIRCLE ( 'NONE', #246, 1.499999999999994449 ) ;
#6090=EDGE_LOOP ( 'NONE', ( #3416, #2700, #3631, #9646 ) ) ;
#6102=VECTOR ( 'NONE', #13630, 1000.000000000000000 ) ;
#6105=EDGE_LOOP ( 'NONE', ( #15297, #6890, #12282, #1004 ) ) ;
#6117=FACE_OUTER_BOUND ( 'NONE', #9490, .T. ) ;
#6119=DIRECTION ( 'NONE',  ( -0.000000000000000000, 1.000000000000000000, -0.000000000000000000 ) ) ;
#6145=DIRECTION ( 'NONE',  ( 1.000000000000000000, 0.000000000000000000, 0.000000000000000000 ) ) ;
#6150=DIRECTION ( 'NONE',  ( 1.000000000000000000, 0.000000000000000000, 0.000000000000000000 ) ) ;
#6154=ORIENTED_EDGE ( 'NONE', *, *, #14542, .F. ) ;
#6155=CARTESIAN_POINT ( 'NONE',  ( 178.0000000000000853, -178.9449732516916072, -29.32815825124560760 ) ) ;
#6156=LINE ( 'NONE', #3776, #6608 ) ;
#6158=LINE ( 'NONE', #283, #2072 ) ;
#6159=( NAMED_UNIT ( * ) SI_UNIT ( $, .STERADIAN. ) SOLID_ANGLE_UNIT ( ) );
#6164=EDGE_CURVE ( 'NONE', #12750, #15193, #14005, .T. ) ;
#6167=EDGE_CURVE ( 'NONE', #8073, #8771, #15206, .T. ) ;
#6172=ORIENTED_EDGE ( 'NONE', *, *, #5524, .F. ) ;
#6175=ORIENTED_EDGE ( 'NONE', *, *, #15398, .F. ) ;
#6179=ORIENTED_EDGE ( 'NONE', *, *, #714, .F. ) ;
#6180=CARTESIAN_POINT ( 'NONE',  ( 184.0000000000000568, -179.3058001507315566, 74.95141194869098911 ) ) ;
#6184=EDGE_LOOP ( 'NONE', ( #459, #12754, #12544, #10634, #14230, #134, #6628, #4493, #6179, #9902, #13577, #8035, #12192, #8484, #9797, #4098, #8559 ) ) ;
#6185=ORIENTED_EDGE ( 'NONE', *, *, #245, .T. ) ;
#6187=ORIENTED_EDGE ( 'NONE', *, *, #12587, .T. ) ;
#6188=CARTESIAN_POINT ( 'NONE',  ( -70.00000000000000000, -181.3058001507315566, -39.95141194869120937 ) ) ;
#6196=ORIENTED_EDGE ( 'NONE', *, *, #14081, .T. ) ;
#6200=AXIS2_PLACEMENT_3D ( 'NONE', #7527, #12325, #6347 ) ;
#6203=CYLINDRICAL_SURFACE ( 'NONE', #3530, 0.4999999999999996114 ) ;
#6214=VERTEX_POINT ( 'NONE', #12814 ) ;
#6216=CYLINDRICAL_SURFACE ( 'NONE', #3379, 0.5000000000000004441 ) ;
#6220=DIRECTION ( 'NONE',  ( 1.000000000000000000, 0.000000000000000000, 0.000000000000000000 ) ) ;
#6224=FACE_OUTER_BOUND ( 'NONE', #2213, .T. ) ;
#6228=EDGE_CURVE ( 'NONE', #10747, #6953, #9281, .T. ) ;
#6233=DIRECTION ( 'NONE',  ( 1.000000000000000000, 0.000000000000000000, 0.000000000000000000 ) ) ;
#6235=DIRECTION ( 'NONE',  ( 0.000000000000000000, 0.000000000000000000, -1.000000000000000000 ) ) ;
#6237=ORIENTED_EDGE ( 'NONE', *, *, #10181, .T. ) ;
#6242=AXIS2_PLACEMENT_3D ( 'NONE', #2028, #4315, #9155 ) ;
#6246=ADVANCED_FACE ( 'NONE', ( #9437 ), #14158, .T. ) ;
#6250=ORIENTED_EDGE ( 'NONE', *, *, #11695, .F. ) ;
#6251=LINE ( 'NONE', #216, #9414 ) ;
#6252=DIRECTION ( 'NONE',  ( 0.000000000000000000, 1.000000000000000000, 0.000000000000000000 ) ) ;
#6256=VECTOR ( 'NONE', #384, 1000.000000000000000 ) ;
#6266=EDGE_LOOP ( 'NONE', ( #10284, #1450, #1958, #12572, #339 ) ) ;
#6270=CIRCLE ( 'NONE', #11558, 0.5000000000000004441 ) ;
#6271=VERTEX_POINT ( 'NONE', #12972 ) ;
#6273=CARTESIAN_POINT ( 'NONE',  ( -64.00000000000002842, -179.3058001507315566, -30.31842631998718574 ) ) ;
#6274=DIRECTION ( 'NONE',  ( 0.000000000000000000, -0.9902680687415714722, 0.1391731009600582769 ) ) ;
#6278=FILL_AREA_STYLE ('',( #11246 ) ) ;
#6280=VERTEX_POINT ( 'NONE', #6690 ) ;
#6296=AXIS2_PLACEMENT_3D ( 'NONE', #11961, #6119, #7155 ) ;
#6303=EDGE_CURVE ( 'NONE', #13507, #831, #1488, .T. ) ;
#6304=CARTESIAN_POINT ( 'NONE',  ( -61.94838851346079167, 15.53993994372673981, 37.49999999999991473 ) ) ;
#6305=VERTEX_POINT ( 'NONE', #3121 ) ;
#6316=CIRCLE ( 'NONE', #6571, 0.5000000000000004441 ) ;
#6319=ORIENTED_EDGE ( 'NONE', *, *, #7953, .F. ) ;
#6323=VECTOR ( 'NONE', #7092, 1000.000000000000000 ) ;
#6327=ORIENTED_EDGE ( 'NONE', *, *, #5187, .T. ) ;
#6333=CYLINDRICAL_SURFACE ( 'NONE', #8911, 0.5000000000000000000 ) ;
#6334=FACE_OUTER_BOUND ( 'NONE', #7554, .T. ) ;
#6336=EDGE_CURVE ( 'NONE', #4169, #5101, #5540, .T. ) ;
#6338=CARTESIAN_POINT ( 'NONE',  ( -63.50000000000002842, 15.17911304468679745, 25.93769382960995884 ) ) ;
#6339=EDGE_LOOP ( 'NONE', ( #4461, #1487, #2786, #5499 ) ) ;
#6345=CARTESIAN_POINT ( 'NONE',  ( 178.0000000000000853, -179.3058001507315566, 52.76585208085545275 ) ) ;
#6346=VERTEX_POINT ( 'NONE', #1360 ) ;
#6347=DIRECTION ( 'NONE',  ( 0.000000000000000000, 0.000000000000000000, 1.000000000000000000 ) ) ;
#6349=CARTESIAN_POINT ( 'NONE',  ( -76.50000000000001421, 15.03993994372673981, -3.075184203610571654 ) ) ;
#6350=ORIENTED_EDGE ( 'NONE', *, *, #4196, .F. ) ;
#6352=VECTOR ( 'NONE', #8652, 1000.000000000000000 ) ;
#6356=CARTESIAN_POINT ( 'NONE',  ( -76.00000000000001421, 15.03993994372673981, -3.075184203610571654 ) ) ;
#6357=DIRECTION ( 'NONE',  ( 0.000000000000000000, 0.000000000000000000, -1.000000000000000000 ) ) ;
#6359=EDGE_CURVE ( 'NONE', #3126, #592, #12576, .T. ) ;
#6360=ADVANCED_FACE ( 'NONE', ( #6117 ), #8564, .T. ) ;
#6366=CARTESIAN_POINT ( 'NONE',  ( 190.0000000000000853, 21.51947656765315386, 25.04661384777570987 ) ) ;
#6368=FACE_OUTER_BOUND ( 'NONE', #11256, .T. ) ;
#6371=VECTOR ( 'NONE', #8754, 1000.000000000000114 ) ;
#6376=ADVANCED_FACE ( 'NONE', ( #4853 ), #9671, .F. ) ;
#6382=VECTOR ( 'NONE', #2458, 1000.000000000000000 ) ;
#6388=DIRECTION ( 'NONE',  ( 1.000000000000000000, 0.000000000000000000, 0.000000000000000000 ) ) ;
#6391=EDGE_LOOP ( 'NONE', ( #9779, #9057 ) ) ;
#6392=DIRECTION ( 'NONE',  ( 0.000000000000000000, 0.000000000000000000, 1.000000000000000000 ) ) ;
#6396=DIRECTION ( 'NONE',  ( 0.000000000000000000, 0.000000000000000000, 1.000000000000000000 ) ) ;
#6407=AXIS2_PLACEMENT_3D ( 'NONE', #14103, #11755, #7824 ) ;
#6412=VECTOR ( 'NONE', #10619, 1000.000000000000000 ) ;
#6422=MECHANICAL_DESIGN_GEOMETRIC_PRESENTATION_REPRESENTATION('',(#2123),#1619);
#6427=CARTESIAN_POINT ( 'NONE',  ( 190.5000000000000568, 15.53993994372673981, -17.50000000000002487 ) ) ;
#6434=ORIENTED_EDGE ( 'NONE', *, *, #11392, .F. ) ;
#6438=CARTESIAN_POINT ( 'NONE',  ( 177.5000000000000853, 15.03993994372673804, 38.07518420361041933 ) ) ;
#6440=CIRCLE ( 'NONE', #9458, 1.000000000000000888 ) ;
#6443=CARTESIAN_POINT ( 'NONE',  ( 190.5000000000000568, -181.3058001507315566, 84.88378295107885663 ) ) ;
#6444=DIRECTION ( 'NONE',  ( 5.518327896226365911E-17, -0.9902680687415714722, 0.1391731009600582769 ) ) ;
#6447=EDGE_LOOP ( 'NONE', ( #1060, #3190, #10004, #802 ) ) ;
#6450=EDGE_CURVE ( 'NONE', #10552, #3344, #13848, .T. ) ;
#6451=EDGE_CURVE ( 'NONE', #12140, #5020, #15488, .T. ) ;
#6457=CARTESIAN_POINT ( 'NONE',  ( 178.0000000000000853, 16.03993994372673981, 7.553451883674125344E-16 ) ) ;
#6458=DIRECTION ( 'NONE',  ( -0.000000000000000000, -0.000000000000000000, 1.000000000000000000 ) ) ;
#6461=EDGE_CURVE ( 'NONE', #720, #14008, #11088, .T. ) ;
#6462=AXIS2_PLACEMENT_3D ( 'NONE', #1103, #9406, #2214 ) ;
#6464=DIRECTION ( 'NONE',  ( 0.000000000000000000, 0.1391731009600592484, 0.9902680687415712502 ) ) ;
#6467=AXIS2_PLACEMENT_3D ( 'NONE', #13039, #892, #5723 ) ;
#6469=EDGE_LOOP ( 'NONE', ( #869, #3477, #6327, #11868 ) ) ;
#6474=LINE ( 'NONE', #1561, #4455 ) ;
#6478=AXIS2_PLACEMENT_3D ( 'NONE', #264, #5250, #1696 ) ;
#6480=DIRECTION ( 'NONE',  ( 0.000000000000000000, 1.734723475976805517E-15, 1.000000000000000000 ) ) ;
#6481=EDGE_CURVE ( 'NONE', #5077, #8326, #12826, .T. ) ;
#6485=FACE_OUTER_BOUND ( 'NONE', #6469, .T. ) ;
#6487=ORIENTED_EDGE ( 'NONE', *, *, #1795, .F. ) ;
#6493=CARTESIAN_POINT ( 'NONE',  ( 177.5000000000000853, 16.03993994372673981, 24.94742576086838781 ) ) ;
#6496=VERTEX_POINT ( 'NONE', #14930 ) ;
#6497=ADVANCED_FACE ( 'NONE', ( #9907 ), #10059, .F. ) ;
#6502=ORIENTED_EDGE ( 'NONE', *, *, #4226, .F. ) ;
#6505=VERTEX_POINT ( 'NONE', #12488 ) ;
#6506=ORIENTED_EDGE ( 'NONE', *, *, #8851, .T. ) ;
#6508=EDGE_CURVE ( 'NONE', #7789, #15483, #8067, .T. ) ;
#6514=LINE ( 'NONE', #10139, #3258 ) ;
#6516=EDGE_CURVE ( 'NONE', #9609, #3320, #1230, .T. ) ;
#6525=CARTESIAN_POINT ( 'NONE',  ( -76.50000000000001421, -181.3058001507315566, 84.88378295107885663 ) ) ;
#6529=ORIENTED_EDGE ( 'NONE', *, *, #6049, .F. ) ;
#6530=CARTESIAN_POINT ( 'NONE',  ( 177.5000000000000853, 16.03993994372673626, 52.49999999999997868 ) ) ;
#6534=CARTESIAN_POINT ( 'NONE',  ( 184.0000000000000568, 17.53993994372673981, -10.99999999999999645 ) ) ;
#6535=EDGE_CURVE ( 'NONE', #6993, #13446, #6514, .T. ) ;
#6536=ADVANCED_FACE ( 'NONE', ( #12333 ), #5276, .T. ) ;
#6550=CARTESIAN_POINT ( 'NONE',  ( -76.00000000000001421, -179.3058001507315566, -51.45141194869120227 ) ) ;
#6555=CARTESIAN_POINT ( 'NONE',  ( 177.5000000000000853, 14.97035339324670744, 37.58005016923963382 ) ) ;
#6558=EDGE_CURVE ( 'NONE', #5784, #14668, #11396, .T. ) ;
#6560=DIRECTION ( 'NONE',  ( 0.000000000000000000, 0.000000000000000000, 1.000000000000000000 ) ) ;
#6564=VECTOR ( 'NONE', #13111, 1000.000000000000000 ) ;
#6571=AXIS2_PLACEMENT_3D ( 'NONE', #1605, #12336, #4048 ) ;
#6572=ORIENTED_EDGE ( 'NONE', *, *, #11020, .F. ) ;
#6575=EDGE_CURVE ( 'NONE', #12789, #12371, #12584, .T. ) ;
#6577=DIRECTION ( 'NONE',  ( 1.000000000000000000, 0.000000000000000000, 0.000000000000000000 ) ) ;
#6578=ORIENTED_EDGE ( 'NONE', *, *, #13242, .F. ) ;
#6579=CIRCLE ( 'NONE', #7080, 1.500000000000001332 ) ;
#6580=AXIS2_PLACEMENT_3D ( 'NONE', #6457, #2971, #7721 ) ;
#6581=PRODUCT_CONTEXT ( 'NONE', #2417, 'mechanical' ) ;
#6582=ORIENTED_EDGE ( 'NONE', *, *, #4444, .F. ) ;
#6588=ORIENTED_EDGE ( 'NONE', *, *, #6167, .F. ) ;
#6591=CARTESIAN_POINT ( 'NONE',  ( 178.0000000000000853, -178.8058001507315566, 52.19066787724494816 ) ) ;
#6592=AXIS2_PLACEMENT_3D ( 'NONE', #13705, #8912, #6388 ) ;
#6597=DIRECTION ( 'NONE',  ( 1.000000000000000000, 0.000000000000000000, 0.000000000000000000 ) ) ;
#6598=CARTESIAN_POINT ( 'NONE',  ( -64.00000000000002842, -179.8058001507315566, 52.49999999999997868 ) ) ;
#6600=DIRECTION ( 'NONE',  ( 0.000000000000000000, -4.956352788505162775E-17, 1.000000000000000000 ) ) ;
#6604=ORIENTED_EDGE ( 'NONE', *, *, #9339, .T. ) ;
#6608=VECTOR ( 'NONE', #5041, 1000.000000000000000 ) ;
#6613=CIRCLE ( 'NONE', #7616, 0.5000000000000004441 ) ;
#6614=EDGE_CURVE ( 'NONE', #9726, #8808, #7578, .T. ) ;
#6615=FACE_OUTER_BOUND ( 'NONE', #8714, .T. ) ;
#6627=CARTESIAN_POINT ( 'NONE',  ( 190.0000000000000568, -179.8058001507315566, -17.50000000000002487 ) ) ;
#6628=ORIENTED_EDGE ( 'NONE', *, *, #8851, .F. ) ;
#6630=DIRECTION ( 'NONE',  ( -1.000000000000000000, 0.000000000000000000, 0.000000000000000000 ) ) ;
#6632=ADVANCED_FACE ( 'NONE', ( #8011 ), #5555, .F. ) ;
#6634=DIRECTION ( 'NONE',  ( 0.000000000000000000, 0.000000000000000000, 1.000000000000000000 ) ) ;
#6636=CIRCLE ( 'NONE', #3340, 0.4999999999999996114 ) ;
#6640=VECTOR ( 'NONE', #15603, 1000.000000000000000 ) ;
#6641=DIRECTION ( 'NONE',  ( 0.000000000000000000, 0.1391731009600660485, -0.9902680687415702510 ) ) ;
#6651=ADVANCED_FACE ( 'NONE', ( #6902 ), #5630, .T. ) ;
#6652=ORIENTED_EDGE ( 'NONE', *, *, #10394, .F. ) ;
#6653=EDGE_CURVE ( 'NONE', #9261, #3488, #5557, .T. ) ;
#6661=AXIS2_PLACEMENT_3D ( 'NONE', #13881, #674, #6784 ) ;
#6662=DIRECTION ( 'NONE',  ( 1.000000000000000000, 0.000000000000000000, 0.000000000000000000 ) ) ;
#6668=ORIENTED_EDGE ( 'NONE', *, *, #14429, .F. ) ;
#6674=AXIS2_PLACEMENT_3D ( 'NONE', #7020, #11828, #11905 ) ;
#6678=VECTOR ( 'NONE', #8900, 1000.000000000000000 ) ;
#6679=CARTESIAN_POINT ( 'NONE',  ( 190.0000000000000853, -179.8058001507315566, 65.31842631998698323 ) ) ;
#6681=ORIENTED_EDGE ( 'NONE', *, *, #14529, .T. ) ;
#6682=CARTESIAN_POINT ( 'NONE',  ( 177.5000000000000853, -178.8058001507315566, -18.19066787724516843 ) ) ;
#6685=DIRECTION ( 'NONE',  ( -1.000000000000000000, -2.751328491981765035E-32, 3.965082230804130220E-16 ) ) ;
#6689=ORIENTED_EDGE ( 'NONE', *, *, #8483, .F. ) ;
#6690=CARTESIAN_POINT ( 'NONE',  ( -64.00000000000002842, 15.53993994372673981, 10.05257423913146475 ) ) ;
#6700=DIRECTION ( 'NONE',  ( -1.000000000000000000, 0.000000000000000000, 0.000000000000000000 ) ) ;
#6705=ORIENTED_EDGE ( 'NONE', *, *, #4008, .T. ) ;
#6714=LINE ( 'NONE', #5441, #2097 ) ;
#6718=DIRECTION ( 'NONE',  ( -1.000000000000000000, 0.000000000000000000, 0.000000000000000000 ) ) ;
#6721=ORIENTED_EDGE ( 'NONE', *, *, #3750, .T. ) ;
#6724=LINE ( 'NONE', #11527, #297 ) ;
#6725=DIRECTION ( 'NONE',  ( 1.000000000000000000, -0.000000000000000000, -0.000000000000000000 ) ) ;
#6728=FACE_OUTER_BOUND ( 'NONE', #568, .T. ) ;
#6729=ORIENTED_EDGE ( 'NONE', *, *, #3664, .F. ) ;
#6737=FACE_OUTER_BOUND ( 'NONE', #10518, .T. ) ;
#6739=VERTEX_POINT ( 'NONE', #2679 ) ;
#6740=EDGE_LOOP ( 'NONE', ( #11161, #2368, #6319, #3311, #8429, #5755 ) ) ;
#6745=CARTESIAN_POINT ( 'NONE',  ( -76.00000000000001421, 15.03993994372673804, 24.94742576086838781 ) ) ;
#6754=ORIENTED_EDGE ( 'NONE', *, *, #14372, .T. ) ;
#6762=EDGE_CURVE ( 'NONE', #1955, #2689, #13551, .T. ) ;
#6772=ORIENTED_EDGE ( 'NONE', *, *, #13850, .F. ) ;
#6774=CIRCLE ( 'NONE', #1203, 0.5000000000000004441 ) ;
#6776=ORIENTED_EDGE ( 'NONE', *, *, #14718, .F. ) ;
#6778=CARTESIAN_POINT ( 'NONE',  ( 190.0000000000000568, -178.8058001507315566, 53.19066787724494816 ) ) ;
#6784=DIRECTION ( 'NONE',  ( 1.000000000000000000, 0.000000000000000000, 0.000000000000000000 ) ) ;
#6786=ORIENTED_EDGE ( 'NONE', *, *, #5460, .F. ) ;
#6788=LINE ( 'NONE', #6947, #12203 ) ;
#6789=CARTESIAN_POINT ( 'NONE',  ( -64.00000000000002842, 15.03993994372673804, 24.94742576086838781 ) ) ;
#6791=ORIENTED_EDGE ( 'NONE', *, *, #14042, .T. ) ;
#6794=DIRECTION ( 'NONE',  ( 1.000000000000000000, 0.000000000000000000, 0.000000000000000000 ) ) ;
#6799=VECTOR ( 'NONE', #15537, 1000.000000000000000 ) ;
#6800=AXIS2_PLACEMENT_3D ( 'NONE', #12807, #1996, #5788 ) ;
#6801=ADVANCED_FACE ( 'NONE', ( #14740 ), #7501, .F. ) ;
#6803=ORIENTED_EDGE ( 'NONE', *, *, #6164, .T. ) ;
#6808=DIRECTION ( 'NONE',  ( 0.000000000000000000, 1.000000000000000000, 0.000000000000000000 ) ) ;
#6810=DIRECTION ( 'NONE',  ( 5.518327896226373307E-17, 0.9902680687415712502, 0.1391731009600586100 ) ) ;
#6813=EDGE_LOOP ( 'NONE', ( #15300, #13743, #7356, #4586 ) ) ;
#6823=DIRECTION ( 'NONE',  ( 0.000000000000000000, 1.000000000000000000, 6.938893903907227145E-17 ) ) ;
#6824=EDGE_CURVE ( 'NONE', #12658, #12750, #11604, .T. ) ;
#6827=FACE_OUTER_BOUND ( 'NONE', #6813, .T. ) ;
#6829=ORIENTED_EDGE ( 'NONE', *, *, #6359, .T. ) ;
#6831=CIRCLE ( 'NONE', #7600, 1.499999999999997780 ) ;
#6834=FACE_OUTER_BOUND ( 'NONE', #11618, .T. ) ;
#6843=CIRCLE ( 'NONE', #4550, 1.000000000000000000 ) ;
#6846=EDGE_LOOP ( 'NONE', ( #13141, #10480, #3449, #4506, #1769, #6350 ) ) ;
#6852=CARTESIAN_POINT ( 'NONE',  ( 190.0000000000000568, 14.97035339324670922, -2.580050169239785696 ) ) ;
#6854=EDGE_LOOP ( 'NONE', ( #1504, #11384, #10934, #13290 ) ) ;
#6868=CIRCLE ( 'NONE', #2582, 1.000000000000000888 ) ;
#6870=CARTESIAN_POINT ( 'NONE',  ( -63.50000000000002842, -178.8058001507315566, -18.19066787724516843 ) ) ;
#6873=CARTESIAN_POINT ( 'NONE',  ( -64.00000000000002842, 15.03993994372673981, -3.075184203610571654 ) ) ;
#6874=ORIENTED_EDGE ( 'NONE', *, *, #13202, .F. ) ;
#6876=PLANE ( 'NONE',  #11039 ) ;
#6878=CIRCLE ( 'NONE', #9894, 0.9999999999999991118 ) ;
#6881=CARTESIAN_POINT ( 'NONE',  ( -64.00000000000002842, -179.8058001507315566, -51.45141194869119516 ) ) ;
#6887=VERTEX_POINT ( 'NONE', #8686 ) ;
#6890=ORIENTED_EDGE ( 'NONE', *, *, #2606, .F. ) ;
#6893=CARTESIAN_POINT ( 'NONE',  ( 178.0000000000000853, -178.6666270497714777, 53.18093594598651919 ) ) ;
#6895=ORIENTED_EDGE ( 'NONE', *, *, #1702, .T. ) ;
#6896=CARTESIAN_POINT ( 'NONE',  ( 178.0000000000000853, -179.3058001507315566, -29.88378295107905913 ) ) ;
#6898=COLOUR_RGB ( '', 0.72549020, 0.75294118, 0.79215686) ;
#6902=FACE_OUTER_BOUND ( 'NONE', #9369, .T. ) ;
#6906=ORIENTED_EDGE ( 'NONE', *, *, #8613, .T. ) ;
#6908=EDGE_CURVE ( 'NONE', #14048, #1178, #1244, .T. ) ;
#6910=LINE ( 'NONE', #10691, #1233 ) ;
#6913=UNCERTAINTY_MEASURE_WITH_UNIT (LENGTH_MEASURE( 1.000000000000000082E-05 ), #248, 'distance_accuracy_value', 'NONE');
#6915=TOROIDAL_SURFACE ( 'NONE', #1347, 1.000000000000000000, 0.5000000000000000000 ) ;
#6916=ORIENTED_EDGE ( 'NONE', *, *, #14912, .T. ) ;
#6928=EDGE_CURVE ( 'NONE', #12140, #11697, #8839, .T. ) ;
#6929=CIRCLE ( 'NONE', #7409, 0.5000000000000004441 ) ;
#6938=CYLINDRICAL_SURFACE ( 'NONE', #9595, 1.499999999999994449 ) ;
#6945=CARTESIAN_POINT ( 'NONE',  ( -76.00000000000001421, -178.6666270497714777, -18.18093594598673945 ) ) ;
#6947=CARTESIAN_POINT ( 'NONE',  ( 177.5000000000000853, -179.3058001507315566, 84.88378295107887084 ) ) ;
#6949=CARTESIAN_POINT ( 'NONE',  ( 190.5000000000000568, -179.3058001507315566, -30.31842631998718574 ) ) ;
#6950=DIRECTION ( 'NONE',  ( 0.000000000000000000, -1.000000000000000000, -4.956352788505162775E-17 ) ) ;
#6952=ORIENTED_EDGE ( 'NONE', *, *, #915, .F. ) ;
#6953=VERTEX_POINT ( 'NONE', #12276 ) ;
#6954=DIRECTION ( 'NONE',  ( 0.000000000000000000, -0.1391731009600582492, -0.9902680687415713612 ) ) ;
#6955=CARTESIAN_POINT ( 'NONE',  ( -76.00000000000004263, -179.3058001507315566, 65.31842631998698323 ) ) ;
#6956=ORIENTED_EDGE ( 'NONE', *, *, #11449, .F. ) ;
#6958=CARTESIAN_POINT ( 'NONE',  ( 190.0000000000000568, 15.03993994372673981, 10.05257423913146475 ) ) ;
#6959=CIRCLE ( 'NONE', #115, 0.5000000000000004441 ) ;
#6965=DIRECTION ( 'NONE',  ( 1.000000000000000000, 2.751328491981765035E-32, -3.965082230804130220E-16 ) ) ;
#6966=ORIENTED_EDGE ( 'NONE', *, *, #4197, .F. ) ;
#6968=VECTOR ( 'NONE', #15204, 1000.000000000000000 ) ;
#6971=VERTEX_POINT ( 'NONE', #10961 ) ;
#6979=EDGE_CURVE ( 'NONE', #1838, #12812, #3284, .T. ) ;
#6982=AXIS2_PLACEMENT_3D ( 'NONE', #11332, #3764, #11029 ) ;
#6983=ORIENTED_EDGE ( 'NONE', *, *, #11908, .T. ) ;
#6990=VERTEX_POINT ( 'NONE', #13224 ) ;
#6993=VERTEX_POINT ( 'NONE', #9617 ) ;
#7005=DIRECTION ( 'NONE',  ( 0.000000000000000000, 0.000000000000000000, 1.000000000000000000 ) ) ;
#7006=DIRECTION ( 'NONE',  ( -1.000000000000000000, -2.751328491981765035E-32, 3.965082230804130220E-16 ) ) ;
#7011=ADVANCED_FACE ( 'NONE', ( #12202 ), #13460, .F. ) ;
#7015=CIRCLE ( 'NONE', #8777, 0.5000000000000000000 ) ;
#7017=EDGE_CURVE ( 'NONE', #1592, #3135, #14413, .T. ) ;
#7020=CARTESIAN_POINT ( 'NONE',  ( 178.0000000000000853, -178.8058001507315566, 52.19066787724494816 ) ) ;
#7024=VECTOR ( 'NONE', #13629, 1000.000000000000000 ) ;
#7027=DIRECTION ( 'NONE',  ( 0.000000000000000000, 0.9902680687415714722, -0.1391731009600582769 ) ) ;
#7029=VERTEX_POINT ( 'NONE', #14487 ) ;
#7030=AXIS2_PLACEMENT_3D ( 'NONE', #15033, #9060, #6464 ) ;
#7032=DIRECTION ( 'NONE',  ( -1.000000000000000000, 0.000000000000000000, 0.000000000000000000 ) ) ;
#7036=FACE_OUTER_BOUND ( 'NONE', #10597, .T. ) ;
#7040=AXIS2_PLACEMENT_3D ( 'NONE', #12117, #5170, #3598 ) ;
#7047=ORIENTED_EDGE ( 'NONE', *, *, #7803, .F. ) ;
#7049=DIRECTION ( 'NONE',  ( 1.000000000000000000, 0.000000000000000000, 0.000000000000000000 ) ) ;
#7057=AXIS2_PLACEMENT_3D ( 'NONE', #1055, #5880, #10698 ) ;
#7060=ORIENTED_EDGE ( 'NONE', *, *, #3199, .F. ) ;
#7061=CARTESIAN_POINT ( 'NONE',  ( -64.00000000000002842, 16.03993994372673981, 38.07518420361041933 ) ) ;
#7065=CARTESIAN_POINT ( 'NONE',  ( 177.5000000000000853, 15.53993994372673804, 24.94742576086838781 ) ) ;
#7067=AXIS2_PLACEMENT_3D ( 'NONE', #10320, #8987, #7729 ) ;
#7080=AXIS2_PLACEMENT_3D ( 'NONE', #15119, #832, #9152 ) ;
#7084=VERTEX_POINT ( 'NONE', #5335 ) ;
#7088=CARTESIAN_POINT ( 'NONE',  ( 190.5000000000000568, 15.17911304468679923, 9.062306170389897275 ) ) ;
#7090=ORIENTED_EDGE ( 'NONE', *, *, #164, .F. ) ;
#7091=ORIENTED_EDGE ( 'NONE', *, *, #7158, .F. ) ;
#7092=DIRECTION ( 'NONE',  ( 1.000000000000000000, -0.000000000000000000, -0.000000000000000000 ) ) ;
#7096=DIRECTION ( 'NONE',  ( -1.000000000000000000, 0.000000000000000000, 0.000000000000000000 ) ) ;
#7097=FACE_OUTER_BOUND ( 'NONE', #7264, .T. ) ;
#7101=ADVANCED_FACE ( 'NONE', ( #7880 ), #12358, .T. ) ;
#7104=CARTESIAN_POINT ( 'NONE',  ( 178.0000000000000853, -178.8753867012115961, -29.82329228561640022 ) ) ;
#7105=AXIS2_PLACEMENT_3D ( 'NONE', #5092, #3514, #8351 ) ;
#7106=DIRECTION ( 'NONE',  ( -1.000000000000000000, 0.000000000000000000, 0.000000000000000000 ) ) ;
#7110=ORIENTED_EDGE ( 'NONE', *, *, #2606, .T. ) ;
#7123=FACE_OUTER_BOUND ( 'NONE', #9277, .T. ) ;
#7126=AXIS2_PLACEMENT_3D ( 'NONE', #3696, #5120, #7349 ) ;
#7138=CIRCLE ( 'NONE', #5865, 0.5000000000000001110 ) ;
#7146=CYLINDRICAL_SURFACE ( 'NONE', #3507, 1.499999999999994449 ) ;
#7152=AXIS2_PLACEMENT_3D ( 'NONE', #4415, #14043, #3234 ) ;
#7155=DIRECTION ( 'NONE',  ( 0.000000000000000000, 0.000000000000000000, -1.000000000000000000 ) ) ;
#7158=EDGE_CURVE ( 'NONE', #10500, #14360, #581, .T. ) ;
#7160=ADVANCED_FACE ( 'NONE', ( #6615 ), #2796, .T. ) ;
#7172=DIRECTION ( 'NONE',  ( -3.965082230804130220E-16, 0.000000000000000000, 1.000000000000000000 ) ) ;
#7175=VERTEX_POINT ( 'NONE', #13613 ) ;
#7178=FACE_OUTER_BOUND ( 'NONE', #7407, .T. ) ;
#7179=DIRECTION ( 'NONE',  ( 0.000000000000000000, -0.1391731009600582492, -0.9902680687415713612 ) ) ;
#7181=DIRECTION ( 'NONE',  ( 0.000000000000000000, 0.000000000000000000, -1.000000000000000000 ) ) ;
#7183=EDGE_CURVE ( 'NONE', #12077, #11157, #496, .T. ) ;
#7188=CARTESIAN_POINT ( 'NONE',  ( -64.00000000000002842, 13.40307322461931072, 37.29540324609171620 ) ) ;
#7190=FACE_OUTER_BOUND ( 'NONE', #7283, .T. ) ;
#7194=AXIS2_PLACEMENT_3D ( 'NONE', #2193, #2035, #15359 ) ;
#7200=CARTESIAN_POINT ( 'NONE',  ( 177.5000000000000853, 16.03993994372673981, -17.50000000000002487 ) ) ;
#7203=VERTEX_POINT ( 'NONE', #15181 ) ;
#7205=VERTEX_POINT ( 'NONE', #3278 ) ;
#7211=EDGE_LOOP ( 'NONE', ( #12829, #14920, #8765, #13726 ) ) ;
#7214=ORIENTED_EDGE ( 'NONE', *, *, #11456, .T. ) ;
#7218=EDGE_CURVE ( 'NONE', #10763, #13859, #3299, .T. ) ;
#7219=EDGE_CURVE ( 'NONE', #7650, #9167, #814, .T. ) ;
#7220=VECTOR ( 'NONE', #8869, 1000.000000000000114 ) ;
#7221=ORIENTED_EDGE ( 'NONE', *, *, #11318, .T. ) ;
#7226=CYLINDRICAL_SURFACE ( 'NONE', #2920, 0.5000000000000004441 ) ;
#7229=ORIENTED_EDGE ( 'NONE', *, *, #6028, .T. ) ;
#7233=ORIENTED_EDGE ( 'NONE', *, *, #3867, .F. ) ;
#7236=CARTESIAN_POINT ( 'NONE',  ( 177.5000000000000853, -178.6666270497714777, -18.18093594598675011 ) ) ;
#7250=ORIENTED_EDGE ( 'NONE', *, *, #8363, .F. ) ;
#7252=DIRECTION ( 'NONE',  ( 1.000000000000000000, 0.000000000000000000, 0.000000000000000000 ) ) ;
#7253=DIRECTION ( 'NONE',  ( 0.000000000000000000, 0.000000000000000000, 1.000000000000000000 ) ) ;
#7254=EDGE_CURVE ( 'NONE', #815, #4028, #11570, .T. ) ;
#7255=CARTESIAN_POINT ( 'NONE',  ( 178.0000000000000853, 15.53993994372673804, 24.94742576086838781 ) ) ;
#7257=DIRECTION ( 'NONE',  ( 0.000000000000000000, 0.000000000000000000, 1.000000000000000000 ) ) ;
#7262=FACE_BOUND ( 'NONE', #8493, .T. ) ;
#7264=EDGE_LOOP ( 'NONE', ( #4870, #89, #12730, #14315 ) ) ;
#7268=CARTESIAN_POINT ( 'NONE',  ( -64.00000000000002842, -178.7362136002515172, 52.68580191161573367 ) ) ;
#7276=AXIS2_PLACEMENT_3D ( 'NONE', #12602, #1865, #3068 ) ;
#7283=EDGE_LOOP ( 'NONE', ( #12532, #7214, #767, #8210 ) ) ;
#7285=CARTESIAN_POINT ( 'NONE',  ( 175.9483885134608272, -178.8058001507315566, 52.69066787724494816 ) ) ;
#7287=ADVANCED_FACE ( 'NONE', ( #11729 ), #7557, .T. ) ;
#7288=VERTEX_POINT ( 'NONE', #4613 ) ;
#7290=CARTESIAN_POINT ( 'NONE',  ( -76.50000000000004263, -179.8058001507315566, 52.19066787724494816 ) ) ;
#7292=CARTESIAN_POINT ( 'NONE',  ( -76.50000000000004263, 16.03993994372673626, 37.49999999999991473 ) ) ;
#7296=CARTESIAN_POINT ( 'NONE',  ( -70.00000000000000000, -201.3058001507315566, -41.45141194869120227 ) ) ;
#7297=EDGE_CURVE ( 'NONE', #3756, #12140, #10063, .T. ) ;
#7300=CARTESIAN_POINT ( 'NONE',  ( 177.5000000000000853, 16.03993994372673626, 38.07518420361041933 ) ) ;
#7302=VERTEX_POINT ( 'NONE', #8265 ) ;
#7309=AXIS2_PLACEMENT_3D ( 'NONE', #6356, #2954, #7773 ) ;
#7314=SURFACE_STYLE_FILL_AREA ( #6278 ) ;
#7318=CARTESIAN_POINT ( 'NONE',  ( 190.0000000000001137, -178.8058001507315566, 65.31842631998698323 ) ) ;
#7319=DIRECTION ( 'NONE',  ( 0.000000000000000000, 1.734723475976805517E-15, 1.000000000000000000 ) ) ;
#7322=CARTESIAN_POINT ( 'NONE',  ( -76.50000000000001421, 17.53993994372673981, -17.50000000000002487 ) ) ;
#7323=ORIENTED_EDGE ( 'NONE', *, *, #14726, .F. ) ;
#7326=ADVANCED_FACE ( 'NONE', ( #14007, #10387 ), #5882, .F. ) ;
#7328=EDGE_CURVE ( 'NONE', #12014, #8771, #7392, .T. ) ;
#7332=FACE_OUTER_BOUND ( 'NONE', #5782, .T. ) ;
#7334=AXIS2_PLACEMENT_3D ( 'NONE', #11784, #951, #15394 ) ;
#7336=CIRCLE ( 'NONE', #495, 0.5000000000000004441 ) ;
#7337=VECTOR ( 'NONE', #4877, 1000.000000000000000 ) ;
#7339=DIRECTION ( 'NONE',  ( 0.000000000000000000, -0.1391731009600592484, -0.9902680687415712502 ) ) ;
#7340=EDGE_CURVE ( 'NONE', #7302, #12019, #3826, .T. ) ;
#7341=DIRECTION ( 'NONE',  ( 0.000000000000000000, 0.000000000000000000, -1.000000000000000000 ) ) ;
#7342=VECTOR ( 'NONE', #7757, 1000.000000000000000 ) ;
#7343=PLANE ( 'NONE',  #7355 ) ;
#7344=VERTEX_POINT ( 'NONE', #8343 ) ;
#7345=AXIS2_PLACEMENT_3D ( 'NONE', #15302, #4501, #3404 ) ;
#7349=DIRECTION ( 'NONE',  ( 0.000000000000000000, 0.000000000000000000, -1.000000000000000000 ) ) ;
#7355=AXIS2_PLACEMENT_3D ( 'NONE', #12059, #5112, #1236 ) ;
#7356=ORIENTED_EDGE ( 'NONE', *, *, #12725, .F. ) ;
#7357=VECTOR ( 'NONE', #9065, 1000.000000000000000 ) ;
#7359=ORIENTED_EDGE ( 'NONE', *, *, #3199, .T. ) ;
#7374=AXIS2_PLACEMENT_3D ( 'NONE', #1062, #4773, #15335 ) ;
#7375=ORIENTED_EDGE ( 'NONE', *, *, #5440, .F. ) ;
#7377=AXIS2_PLACEMENT_3D ( 'NONE', #6873, #14418, #3616 ) ;
#7379=CARTESIAN_POINT ( 'NONE',  ( 177.5000000000000853, -178.6666270497714777, 53.18093594598651919 ) ) ;
#7383=ORIENTED_EDGE ( 'NONE', *, *, #2749, .T. ) ;
#7389=CARTESIAN_POINT ( 'NONE',  ( 184.0000000000000568, -179.3058001507315566, 76.45141194869098911 ) ) ;
#7392=LINE ( 'NONE', #12183, #2243 ) ;
#7393=ORIENTED_EDGE ( 'NONE', *, *, #14218, .F. ) ;
#7397=ORIENTED_EDGE ( 'NONE', *, *, #9435, .T. ) ;
#7398=CARTESIAN_POINT ( 'NONE',  ( -63.50000000000002842, -178.6666270497714777, 53.18093594598651919 ) ) ;
#7399=DIRECTION ( 'NONE',  ( -3.965082230804130220E-16, 0.000000000000000000, 1.000000000000000000 ) ) ;
#7404=CIRCLE ( 'NONE', #5620, 1.499999999999994449 ) ;
#7407=EDGE_LOOP ( 'NONE', ( #6196, #2633, #12833, #8617 ) ) ;
#7409=AXIS2_PLACEMENT_3D ( 'NONE', #10194, #6725, #11375 ) ;
#7419=LINE ( 'NONE', #1235, #3985 ) ;
#7422=ORIENTED_EDGE ( 'NONE', *, *, #4767, .T. ) ;
#7424=DIRECTION ( 'NONE',  ( -1.000000000000000000, -0.000000000000000000, -0.000000000000000000 ) ) ;
#7427=CARTESIAN_POINT ( 'NONE',  ( 178.0000000000000853, 15.10952649420676863, 9.557440204760682789 ) ) ;
#7430=AXIS2_PLACEMENT_3D ( 'NONE', #8666, #14558, #12200 ) ;
#7441=DIRECTION ( 'NONE',  ( 0.000000000000000000, 0.000000000000000000, 1.000000000000000000 ) ) ;
#7442=LINE ( 'NONE', #14291, #14108 ) ;
#7455=VERTEX_POINT ( 'NONE', #2327 ) ;
#7462=AXIS2_PLACEMENT_3D ( 'NONE', #12095, #13503, #3728 ) ;
#7463=AXIS2_PLACEMENT_3D ( 'NONE', #11242, #12105, #13441 ) ;
#7467=VERTEX_POINT ( 'NONE', #7236 ) ;
#7468=DIRECTION ( 'NONE',  ( -0.000000000000000000, -0.000000000000000000, 1.000000000000000000 ) ) ;
#7471=FACE_OUTER_BOUND ( 'NONE', #14129, .T. ) ;
#7478=ADVANCED_FACE ( 'NONE', ( #1437 ), #8497, .T. ) ;
#7480=CARTESIAN_POINT ( 'NONE',  ( -76.00000000000001421, 15.03993994372673804, 24.94742576086838781 ) ) ;
#7486=DIRECTION ( 'NONE',  ( -3.965082230804130220E-16, 0.000000000000000000, 1.000000000000000000 ) ) ;
#7493=DIRECTION ( 'NONE',  ( 0.000000000000000000, -1.000000000000000000, -6.938893903907227145E-17 ) ) ;
#7494=DIRECTION ( 'NONE',  ( 3.965082230804130220E-16, -0.000000000000000000, -1.000000000000000000 ) ) ;
#7499=EDGE_CURVE ( 'NONE', #13870, #11107, #213, .T. ) ;
#7500=EDGE_CURVE ( 'NONE', #10298, #2939, #9076, .T. ) ;
#7501=CYLINDRICAL_SURFACE ( 'NONE', #14854, 1.500000000000001332 ) ;
#7503=EDGE_CURVE ( 'NONE', #13002, #8697, #15102, .T. ) ;
#7506=CARTESIAN_POINT ( 'NONE',  ( 178.0000000000000853, -179.8058001507315566, -30.31842631998718574 ) ) ;
#7508=EDGE_LOOP ( 'NONE', ( #13661, #13253 ) ) ;
#7510=ORIENTED_EDGE ( 'NONE', *, *, #12304, .T. ) ;
#7512=DIRECTION ( 'NONE',  ( 3.965082230804130220E-16, 1.090924371466202084E-47, 1.000000000000000000 ) ) ;
#7518=AXIS2_PLACEMENT_3D ( 'NONE', #2357, #3695, #11994 ) ;
#7519=DIRECTION ( 'NONE',  ( -1.000000000000000000, -0.000000000000000000, -0.000000000000000000 ) ) ;
#7520=ORIENTED_EDGE ( 'NONE', *, *, #2314, .F. ) ;
#7521=AXIS2_PLACEMENT_3D ( 'NONE', #13579, #11383, #461 ) ;
#7526=ORIENTED_EDGE ( 'NONE', *, *, #10428, .F. ) ;
#7527=CARTESIAN_POINT ( 'NONE',  ( -76.00000000000001421, -178.8058001507315566, 52.19066787724494816 ) ) ;
#7529=AXIS2_PLACEMENT_3D ( 'NONE', #6778, #4313, #14022 ) ;
#7533=CARTESIAN_POINT ( 'NONE',  ( -63.50000000000002842, -179.3058001507315566, -17.19066787724516843 ) ) ;
#7535=AXIS2_PLACEMENT_3D ( 'NONE', #501, #587, #12515 ) ;
#7537=DIRECTION ( 'NONE',  ( 0.000000000000000000, 0.1391731009600660485, -0.9902680687415702510 ) ) ;
#7538=CARTESIAN_POINT ( 'NONE',  ( 178.0000000000000853, -179.3058001507315566, 65.31842631998698323 ) ) ;
#7543=SURFACE_SIDE_STYLE ('',( #7314 ) ) ;
#7546=ORIENTED_EDGE ( 'NONE', *, *, #72, .T. ) ;
#7550=CYLINDRICAL_SURFACE ( 'NONE', #1225, 1.499999999999994449 ) ;
#7554=EDGE_LOOP ( 'NONE', ( #7893, #4228, #5298, #5591 ) ) ;
#7557=TOROIDAL_SURFACE ( 'NONE', #12073, 1.000000000000000000, 0.5000000000000000000 ) ;
#7562=AXIS2_PLACEMENT_3D ( 'NONE', #6679, #11484, #8015 ) ;
#7563=FACE_OUTER_BOUND ( 'NONE', #14127, .T. ) ;
#7566=CARTESIAN_POINT ( 'NONE',  ( 178.0000000000000853, 15.03993994372673981, -3.075184203610571654 ) ) ;
#7571=ORIENTED_EDGE ( 'NONE', *, *, #9662, .T. ) ;
#7574=CARTESIAN_POINT ( 'NONE',  ( -76.00000000000001421, 15.53993994372673981, -2.500000000000071054 ) ) ;
#7578=CIRCLE ( 'NONE', #8580, 0.5000000000000004441 ) ;
#7580=DIRECTION ( 'NONE',  ( -3.965082230804130220E-16, 4.956352788505162775E-17, -1.000000000000000000 ) ) ;
#7584=ORIENTED_EDGE ( 'NONE', *, *, #549, .T. ) ;
#7585=VECTOR ( 'NONE', #12164, 1000.000000000000000 ) ;
#7586=VECTOR ( 'NONE', #6718, 1000.000000000000000 ) ;
#7588=AXIS2_PLACEMENT_3D ( 'NONE', #11984, #1154, #7257 ) ;
#7593=ORIENTED_EDGE ( 'NONE', *, *, #10181, .F. ) ;
#7599=AXIS2_PLACEMENT_3D ( 'NONE', #4026, #14983, #7679 ) ;
#7600=AXIS2_PLACEMENT_3D ( 'NONE', #13541, #2747, #8678 ) ;
#7601=CARTESIAN_POINT ( 'NONE',  ( -70.00000000000000000, 15.53993994372673626, 47.49999999999997868 ) ) ;
#7604=ORIENTED_EDGE ( 'NONE', *, *, #8947, .F. ) ;
#7606=ADVANCED_FACE ( 'NONE', ( #242 ), #1503, .T. ) ;
#7607=CARTESIAN_POINT ( 'NONE',  ( 190.5000000000000853, 16.03993994372673626, 38.07518420361041933 ) ) ;
#7610=ORIENTED_EDGE ( 'NONE', *, *, #203, .T. ) ;
#7611=FACE_OUTER_BOUND ( 'NONE', #12367, .T. ) ;
#7613=FACE_OUTER_BOUND ( 'NONE', #2791, .T. ) ;
#7614=ORIENTED_EDGE ( 'NONE', *, *, #10764, .F. ) ;
#7616=AXIS2_PLACEMENT_3D ( 'NONE', #7318, #11096, #4937 ) ;
#7619=VERTEX_POINT ( 'NONE', #2879 ) ;
#7623=DIRECTION ( 'NONE',  ( 0.000000000000000000, -0.9902680687415702510, 0.1391731009600660485 ) ) ;
#7627=ORIENTED_EDGE ( 'NONE', *, *, #7017, .T. ) ;
#7631=DIRECTION ( 'NONE',  ( 0.000000000000000000, 0.000000000000000000, 1.000000000000000000 ) ) ;
#7634=TOROIDAL_SURFACE ( 'NONE', #7374, 1.000000000000000000, 0.5000000000000000000 ) ;
#7637=CARTESIAN_POINT ( 'NONE',  ( -76.50000000000001421, -179.8058001507315566, -29.88378295107906624 ) ) ;
#7639=EDGE_CURVE ( 'NONE', #2454, #11537, #6316, .T. ) ;
#7640=EDGE_CURVE ( 'NONE', #13140, #234, #9090, .T. ) ;
#7641=DIRECTION ( 'NONE',  ( 1.000000000000000000, 2.751328491981765035E-32, -3.965082230804130220E-16 ) ) ;
#7645=EDGE_LOOP ( 'NONE', ( #11145, #6578, #3628, #13347 ) ) ;
#7648=DIRECTION ( 'NONE',  ( 0.000000000000000000, -1.000000000000000000, 0.000000000000000000 ) ) ;
#7650=VERTEX_POINT ( 'NONE', #11243 ) ;
#7661=CIRCLE ( 'NONE', #2862, 1.000000000000000888 ) ;
#7666=ADVANCED_FACE ( 'NONE', ( #9911 ), #14700, .T. ) ;
#7671=EDGE_CURVE ( 'NONE', #5101, #4169, #3783, .T. ) ;
#7676=AXIS2_PLACEMENT_3D ( 'NONE', #10882, #9615, #8364 ) ;
#7678=DIRECTION ( 'NONE',  ( -1.000000000000000000, 0.000000000000000000, 0.000000000000000000 ) ) ;
#7679=DIRECTION ( 'NONE',  ( 0.000000000000000000, -0.1391731009600592484, 0.9902680687415712502 ) ) ;
#7683=AXIS2_PLACEMENT_3D ( 'NONE', #11074, #9657, #9975 ) ;
#7696=VERTEX_POINT ( 'NONE', #400 ) ;
#7716=VERTEX_POINT ( 'NONE', #5633 ) ;
#7719=CARTESIAN_POINT ( 'NONE',  ( 190.5000000000000568, -179.8058001507315566, -30.31842631998718574 ) ) ;
#7721=DIRECTION ( 'NONE',  ( 0.000000000000000000, -1.000000000000000000, -4.956352788505160310E-17 ) ) ;
#7722=EDGE_CURVE ( 'NONE', #9726, #11537, #14064, .T. ) ;
#7723=CYLINDRICAL_SURFACE ( 'NONE', #14707, 0.5000000000000004441 ) ;
#7724=ORIENTED_EDGE ( 'NONE', *, *, #1967, .T. ) ;
#7726=AXIS2_PLACEMENT_3D ( 'NONE', #463, #14997, #3167 ) ;
#7728=CARTESIAN_POINT ( 'NONE',  ( 177.5000000000000853, -178.9449732516916072, -29.32815825124560760 ) ) ;
#7729=DIRECTION ( 'NONE',  ( 0.000000000000000000, 0.000000000000000000, -1.000000000000000000 ) ) ;
#7732=FACE_OUTER_BOUND ( 'NONE', #13589, .T. ) ;
#7735=ORIENTED_EDGE ( 'NONE', *, *, #2749, .F. ) ;
#7736=CARTESIAN_POINT ( 'NONE',  ( -63.50000000000002842, 15.53993994372673981, -17.50000000000002487 ) ) ;
#7740=PLANE ( 'NONE',  #4699 ) ;
#7743=ORIENTED_EDGE ( 'NONE', *, *, #8190, .F. ) ;
#7749=ORIENTED_EDGE ( 'NONE', *, *, #15382, .T. ) ;
#7754=DIRECTION ( 'NONE',  ( 3.965082230804130220E-16, 1.090924371466202084E-47, 1.000000000000000000 ) ) ;
#7757=DIRECTION ( 'NONE',  ( -1.000000000000000000, 0.000000000000000000, 0.000000000000000000 ) ) ;
#7758=CARTESIAN_POINT ( 'NONE',  ( 184.0000000000000568, 15.53993994372673626, 48.99999999999997158 ) ) ;
#7761=LINE ( 'NONE', #6345, #6256 ) ;
#7764=EDGE_CURVE ( 'NONE', #8197, #3561, #10344, .T. ) ;
#7766=EDGE_LOOP ( 'NONE', ( #6250, #14034, #14617, #1663, #7090, #8941, #4738, #10126, #2020 ) ) ;
#7768=FACE_OUTER_BOUND ( 'NONE', #2910, .T. ) ;
#7769=FACE_OUTER_BOUND ( 'NONE', #8226, .T. ) ;
#7773=DIRECTION ( 'NONE',  ( -3.965082230804130220E-16, 1.090924371466202084E-47, 1.000000000000000000 ) ) ;
#7777=EDGE_CURVE ( 'NONE', #2984, #6971, #10083, .T. ) ;
#7780=AXIS2_PLACEMENT_3D ( 'NONE', #4423, #10671, #15386 ) ;
#7781=ORIENTED_EDGE ( 'NONE', *, *, #12145, .T. ) ;
#7782=DIRECTION ( 'NONE',  ( 0.000000000000000000, 0.000000000000000000, -1.000000000000000000 ) ) ;
#7783=CARTESIAN_POINT ( 'NONE',  ( -63.50000000000002842, 16.03993994372673981, -17.50000000000002487 ) ) ;
#7784=VECTOR ( 'NONE', #5189, 1000.000000000000000 ) ;
#7789=VERTEX_POINT ( 'NONE', #10605 ) ;
#7796=CARTESIAN_POINT ( 'NONE',  ( 177.5000000000000853, 16.03993994372673981, 25.38206912977649665 ) ) ;
#7799=CARTESIAN_POINT ( 'NONE',  ( 190.0000000000000853, -179.3058001507315566, 65.31842631998698323 ) ) ;
#7801=DIRECTION ( 'NONE',  ( 2.751328491981765035E-32, -1.000000000000000000, -1.090924371466202084E-47 ) ) ;
#7803=EDGE_CURVE ( 'NONE', #12658, #138, #11637, .T. ) ;
#7804=EDGE_CURVE ( 'NONE', #13575, #592, #12853, .T. ) ;
#7808=AXIS2_PLACEMENT_3D ( 'NONE', #1956, #6794, #3002 ) ;
#7811=DIRECTION ( 'NONE',  ( -3.965082230804130220E-16, 0.000000000000000000, -1.000000000000000000 ) ) ;
#7814=ORIENTED_EDGE ( 'NONE', *, *, #7804, .T. ) ;
#7818=CARTESIAN_POINT ( 'NONE',  ( -76.00000000000001421, -178.8058001507315566, -30.31842631998718574 ) ) ;
#7824=DIRECTION ( 'NONE',  ( 0.000000000000000000, 0.000000000000000000, -1.000000000000000000 ) ) ;
#7830=AXIS2_PLACEMENT_3D ( 'NONE', #5404, #15015, #13678 ) ;
#7831=VECTOR ( 'NONE', #559, 1000.000000000000114 ) ;
#7833=ORIENTED_EDGE ( 'NONE', *, *, #8001, .F. ) ;
#7834=FACE_OUTER_BOUND ( 'NONE', #5239, .T. ) ;
#7835=DIRECTION ( 'NONE',  ( 0.000000000000000000, 0.000000000000000000, -1.000000000000000000 ) ) ;
#7836=AXIS2_PLACEMENT_3D ( 'NONE', #6598, #1522, #11172 ) ;
#7839=DIRECTION ( 'NONE',  ( 0.000000000000000000, 0.000000000000000000, 1.000000000000000000 ) ) ;
#7841=VECTOR ( 'NONE', #2876, 1000.000000000000000 ) ;
#7849=LINE ( 'NONE', #12636, #2147 ) ;
#7861=DIRECTION ( 'NONE',  ( 3.965082230804130220E-16, 0.000000000000000000, -1.000000000000000000 ) ) ;
#7867=ORIENTED_EDGE ( 'NONE', *, *, #5084, .F. ) ;
#7878=CARTESIAN_POINT ( 'NONE',  ( -61.94838851346079167, -178.8058001507315566, 65.31842631998698323 ) ) ;
#7880=FACE_OUTER_BOUND ( 'NONE', #4425, .T. ) ;
#7881=EDGE_CURVE ( 'NONE', #8586, #1592, #14675, .T. ) ;
#7883=ORIENTED_EDGE ( 'NONE', *, *, #715, .F. ) ;
#7884=AXIS2_PLACEMENT_3D ( 'NONE', #7506, #10029, #5281 ) ;
#7885=CARTESIAN_POINT ( 'NONE',  ( -63.50000000000002842, 16.03993994372673981, -3.075184203610571654 ) ) ;
#7888=CIRCLE ( 'NONE', #10386, 1.000000000000000888 ) ;
#7893=ORIENTED_EDGE ( 'NONE', *, *, #8236, .T. ) ;
#7902=LINE ( 'NONE', #6555, #6968 ) ;
#7903=AXIS2_PLACEMENT_3D ( 'NONE', #798, #9117, #5558 ) ;
#7906=CARTESIAN_POINT ( 'NONE',  ( 177.5000000000000853, 15.60952649420677041, 9.122796835852554409 ) ) ;
#7907=CARTESIAN_POINT ( 'NONE',  ( 178.0000000000000853, -178.8058001507315566, -17.19066787724516843 ) ) ;
#7909=ORIENTED_EDGE ( 'NONE', *, *, #2766, .F. ) ;
#7910=ORIENTED_EDGE ( 'NONE', *, *, #2682, .T. ) ;
#7912=CARTESIAN_POINT ( 'NONE',  ( -63.50000000000002842, -179.8058001507315566, -17.19066787724516843 ) ) ;
#7915=DIRECTION ( 'NONE',  ( -0.000000000000000000, 1.000000000000000000, 6.938893903907227145E-17 ) ) ;
#7918=EDGE_LOOP ( 'NONE', ( #10780, #13723, #12286, #1030 ) ) ;
#7921=AXIS2_PLACEMENT_3D ( 'NONE', #11210, #10028, #5128 ) ;
#7925=DIRECTION ( 'NONE',  ( -1.000000000000000000, -0.000000000000000000, -0.000000000000000000 ) ) ;
#7928=ORIENTED_EDGE ( 'NONE', *, *, #72, .F. ) ;
#7951=CARTESIAN_POINT ( 'NONE',  ( -64.00000000000002842, 15.17911304468680100, 9.062306170389884841 ) ) ;
#7953=EDGE_CURVE ( 'NONE', #11614, #10036, #2225, .T. ) ;
#7955=AXIS2_PLACEMENT_3D ( 'NONE', #9289, #9370, #3056 ) ;
#7960=CARTESIAN_POINT ( 'NONE',  ( -70.00000000000000000, 15.53993994372673981, -12.49999999999999289 ) ) ;
#7962=VERTEX_POINT ( 'NONE', #14604 ) ;
#7968=DIRECTION ( 'NONE',  ( 0.000000000000000000, -0.1391731009600592484, 0.9902680687415712502 ) ) ;
#7969=FACE_BOUND ( 'NONE', #2278, .T. ) ;
#7973=DIRECTION ( 'NONE',  ( -0.000000000000000000, -1.000000000000000000, -0.000000000000000000 ) ) ;
#7975=CYLINDRICAL_SURFACE ( 'NONE', #6661, 0.5000000000000004441 ) ;
#7976=FACE_OUTER_BOUND ( 'NONE', #8748, .T. ) ;
#7982=VERTEX_POINT ( 'NONE', #15475 ) ;
#7986=CARTESIAN_POINT ( 'NONE',  ( -76.50000000000001421, -179.8058001507315566, 84.88378295107887084 ) ) ;
#7987=DIRECTION ( 'NONE',  ( 0.000000000000000000, -0.000000000000000000, 1.000000000000000000 ) ) ;
#7988=DIRECTION ( 'NONE',  ( 3.965082230804130220E-16, 4.956352788505162775E-17, -1.000000000000000000 ) ) ;
#7993=DIRECTION ( 'NONE',  ( -1.000000000000000000, 0.000000000000000000, 0.000000000000000000 ) ) ;
#8001=EDGE_CURVE ( 'NONE', #12589, #4389, #1737, .T. ) ;
#8004=VERTEX_POINT ( 'NONE', #5219 ) ;
#8011=FACE_OUTER_BOUND ( 'NONE', #7645, .T. ) ;
#8013=DIRECTION ( 'NONE',  ( 0.000000000000000000, -1.000000000000000000, -6.938893903907227145E-17 ) ) ;
#8015=DIRECTION ( 'NONE',  ( -1.000000000000000000, 0.000000000000000000, 0.000000000000000000 ) ) ;
#8020=ORIENTED_EDGE ( 'NONE', *, *, #10058, .F. ) ;
#8024=ORIENTED_EDGE ( 'NONE', *, *, #12016, .F. ) ;
#8025=CARTESIAN_POINT ( 'NONE',  ( -76.50000000000001421, -178.8753867012115961, 64.82329228561619061 ) ) ;
#8035=ORIENTED_EDGE ( 'NONE', *, *, #14813, .T. ) ;
#8036=DIRECTION ( 'NONE',  ( 0.000000000000000000, -0.1391731009600591096, 0.9902680687415711391 ) ) ;
#8039=CARTESIAN_POINT ( 'NONE',  ( 0.000000000000000000, 15.03993994372673981, 10.05257423913146475 ) ) ;
#8041=ORIENTED_EDGE ( 'NONE', *, *, #4864, .F. ) ;
#8042=FACE_OUTER_BOUND ( 'NONE', #787, .T. ) ;
#8043=AXIS2_PLACEMENT_3D ( 'NONE', #2060, #10599, #8170 ) ;
#8046=DIRECTION ( 'NONE',  ( 1.000000000000000000, 0.000000000000000000, 0.000000000000000000 ) ) ;
#8047=DIRECTION ( 'NONE',  ( -0.000000000000000000, -0.9902680687415710281, 0.1391731009600611635 ) ) ;
#8053=CARTESIAN_POINT ( 'NONE',  ( 178.0000000000000853, -178.8058001507315566, 52.19066787724494816 ) ) ;
#8054=VECTOR ( 'NONE', #7049, 1000.000000000000000 ) ;
#8055=FACE_OUTER_BOUND ( 'NONE', #12520, .T. ) ;
#8063=ORIENTED_EDGE ( 'NONE', *, *, #5038, .T. ) ;
#8064=FACE_OUTER_BOUND ( 'NONE', #466, .T. ) ;
#8067=CIRCLE ( 'NONE', #14088, 1.499999999999994449 ) ;
#8068=CARTESIAN_POINT ( 'NONE',  ( 190.0000000000000568, 15.03993994372673981, 10.05257423913146475 ) ) ;
#8069=DIRECTION ( 'NONE',  ( 0.000000000000000000, -3.469446951953611033E-15, 1.000000000000000000 ) ) ;
#8071=AXIS2_PLACEMENT_3D ( 'NONE', #7, #8713, #2466 ) ;
#8073=VERTEX_POINT ( 'NONE', #6338 ) ;
#8075=VECTOR ( 'NONE', #9380, 1000.000000000000000 ) ;
#8082=VERTEX_POINT ( 'NONE', #7758 ) ;
#8083=CARTESIAN_POINT ( 'NONE',  ( 178.0000000000000853, 15.03993994372673804, 38.07518420361041933 ) ) ;
#8091=EDGE_LOOP ( 'NONE', ( #664, #2459 ) ) ;
#8096=FACE_OUTER_BOUND ( 'NONE', #13480, .T. ) ;
#8098=EDGE_CURVE ( 'NONE', #13426, #7619, #12167, .T. ) ;
#8099=EDGE_CURVE ( 'NONE', #12671, #14171, #14682, .T. ) ;
#8103=ORIENTED_EDGE ( 'NONE', *, *, #13771, .T. ) ;
#8108=DIRECTION ( 'NONE',  ( -3.965082230804130220E-16, 1.090924371466202084E-47, 1.000000000000000000 ) ) ;
#8120=ORIENTED_EDGE ( 'NONE', *, *, #8624, .F. ) ;
#8124=DIRECTION ( 'NONE',  ( 1.000000000000000000, -2.751328491981765035E-32, 3.965082230804130220E-16 ) ) ;
#8129=ADVANCED_FACE ( 'NONE', ( #8940 ), #8704, .F. ) ;
#8131=CIRCLE ( 'NONE', #7105, 0.4999999999999996114 ) ;
#8134=ADVANCED_FACE ( 'NONE', ( #2699, #12317, #1498 ), #13734, .T. ) ;
#8139=AXIS2_PLACEMENT_3D ( 'NONE', #10472, #13775, #15259 ) ;
#8140=DIRECTION ( 'NONE',  ( 0.000000000000000000, 0.000000000000000000, 1.000000000000000000 ) ) ;
#8142=DIRECTION ( 'NONE',  ( -1.000000000000000000, -2.751328491981765035E-32, 3.965082230804130220E-16 ) ) ;
#8147=DIRECTION ( 'NONE',  ( 0.000000000000000000, 0.000000000000000000, 1.000000000000000000 ) ) ;
#8151=DIRECTION ( 'NONE',  ( 0.000000000000000000, 0.000000000000000000, -1.000000000000000000 ) ) ;
#8154=FILL_AREA_STYLE_COLOUR ( '', #6898 ) ;
#8157=EDGE_CURVE ( 'NONE', #10340, #427, #7138, .T. ) ;
#8161=ADVANCED_FACE ( 'NONE', ( #13574 ), #2779, .F. ) ;
#8162=DIRECTION ( 'NONE',  ( 0.000000000000000000, 0.000000000000000000, 1.000000000000000000 ) ) ;
#8169=ORIENTED_EDGE ( 'NONE', *, *, #2443, .F. ) ;
#8170=DIRECTION ( 'NONE',  ( 0.000000000000000000, 0.000000000000000000, 1.000000000000000000 ) ) ;
#8171=DIRECTION ( 'NONE',  ( 0.000000000000000000, 0.000000000000000000, 1.000000000000000000 ) ) ;
#8181=DIRECTION ( 'NONE',  ( 1.000000000000000000, 2.751328491981765035E-32, -3.965082230804130220E-16 ) ) ;
#8186=UNCERTAINTY_MEASURE_WITH_UNIT (LENGTH_MEASURE( 1.000000000000000082E-05 ), #3150, 'distance_accuracy_value', 'NONE');
#8190=EDGE_CURVE ( 'NONE', #12405, #176, #7404, .T. ) ;
#8193=DIRECTION ( 'NONE',  ( -1.000000000000000000, 0.000000000000000000, 3.965082230804112963E-16 ) ) ;
#8195=ADVANCED_FACE ( 'NONE', ( #6728 ), #9095, .F. ) ;
#8197=VERTEX_POINT ( 'NONE', #10349 ) ;
#8198=CIRCLE ( 'NONE', #7683, 0.5000000000000004441 ) ;
#8199=CARTESIAN_POINT ( 'NONE',  ( 190.5000000000000853, 16.03993994372673981, 24.94742576086838781 ) ) ;
#8201=VERTEX_POINT ( 'NONE', #9325 ) ;
#8203=TOROIDAL_SURFACE ( 'NONE', #12456, 1.000000000000000000, 0.5000000000000000000 ) ;
#8209=ORIENTED_EDGE ( 'NONE', *, *, #3824, .F. ) ;
#8210=ORIENTED_EDGE ( 'NONE', *, *, #12398, .T. ) ;
#8211=CARTESIAN_POINT ( 'NONE',  ( 184.0000000000000568, 15.53993994372673626, 47.49999999999997868 ) ) ;
#8212=CARTESIAN_POINT ( 'NONE',  ( 178.0000000000000853, 15.53993994372673626, 52.49999999999997868 ) ) ;
#8213=AXIS2_PLACEMENT_3D ( 'NONE', #2012, #5732, #1855 ) ;
#8220=DIRECTION ( 'NONE',  ( 1.000000000000000000, 0.000000000000000000, 0.000000000000000000 ) ) ;
#8221=EDGE_CURVE ( 'NONE', #6887, #101, #11612, .T. ) ;
#8223=DIRECTION ( 'NONE',  ( 1.000000000000000000, 0.000000000000000000, 3.965082230804112963E-16 ) ) ;
#8224=CARTESIAN_POINT ( 'NONE',  ( -64.00000000000002842, -178.8058001507315566, -17.19066787724516843 ) ) ;
#8226=EDGE_LOOP ( 'NONE', ( #7383, #4309, #4608, #8945, #154 ) ) ;
#8228=DIRECTION ( 'NONE',  ( -0.000000000000000000, -0.000000000000000000, -1.000000000000000000 ) ) ;
#8231=DIRECTION ( 'NONE',  ( -1.000000000000000000, -2.751328491981765035E-32, 3.965082230804130220E-16 ) ) ;
#8232=LINE ( 'NONE', #13009, #11870 ) ;
#8234=VERTEX_POINT ( 'NONE', #777 ) ;
#8236=EDGE_CURVE ( 'NONE', #12968, #7962, #1583, .T. ) ;
#8237=CYLINDRICAL_SURFACE ( 'NONE', #14407, 0.5000000000000001110 ) ;
#8245=DIRECTION ( 'NONE',  ( -3.965082230804130220E-16, 4.956352788505162775E-17, -1.000000000000000000 ) ) ;
#8249=AXIS2_PLACEMENT_3D ( 'NONE', #12993, #10960, #3527 ) ;
#8255=DIRECTION ( 'NONE',  ( 0.000000000000000000, 4.956352788505162775E-17, -1.000000000000000000 ) ) ;
#8258=ORIENTED_EDGE ( 'NONE', *, *, #364, .T. ) ;
#8262=DIRECTION ( 'NONE',  ( 0.000000000000000000, 1.000000000000000000, -0.000000000000000000 ) ) ;
#8263=DIRECTION ( 'NONE',  ( 0.000000000000000000, -0.1391731009600592484, 0.9902680687415712502 ) ) ;
#8264=EDGE_CURVE ( 'NONE', #5867, #5228, #9669, .T. ) ;
#8265=CARTESIAN_POINT ( 'NONE',  ( -76.00000000000001421, 15.53993994372673981, -3.075184203610571654 ) ) ;
#8266=ORIENTED_EDGE ( 'NONE', *, *, #7158, .T. ) ;
#8275=CARTESIAN_POINT ( 'NONE',  ( -76.50000000000001421, 15.47035339324671099, -2.004865965629286872 ) ) ;
#8283=CARTESIAN_POINT ( 'NONE',  ( -64.00000000000002842, 15.03993994372673804, 24.94742576086838781 ) ) ;
#8284=CARTESIAN_POINT ( 'NONE',  ( -63.50000000000002842, -181.3058001507315566, 84.88378295107885663 ) ) ;
#8290=EDGE_CURVE ( 'NONE', #3756, #2220, #4154, .T. ) ;
#8292=DIRECTION ( 'NONE',  ( 3.965082230804130220E-16, 1.090924371466202084E-47, 1.000000000000000000 ) ) ;
#8293=CARTESIAN_POINT ( 'NONE',  ( -76.00000000000001421, 16.03993994372673981, -7.458121719691109004E-14 ) ) ;
#8294=AXIS2_PLACEMENT_3D ( 'NONE', #4431, #14059, #2143 ) ;
#8295=DIRECTION ( 'NONE',  ( 0.000000000000000000, 0.9902680687415714722, -0.1391731009600582769 ) ) ;
#8302=CARTESIAN_POINT ( 'NONE',  ( -76.50000000000001421, 15.53993994372673981, -17.50000000000002487 ) ) ;
#8305=EDGE_CURVE ( 'NONE', #2220, #7302, #12521, .T. ) ;
#8308=ORIENTED_EDGE ( 'NONE', *, *, #11695, .T. ) ;
#8310=VERTEX_POINT ( 'NONE', #14803 ) ;
#8315=ORIENTED_EDGE ( 'NONE', *, *, #7503, .F. ) ;
#8316=TOROIDAL_SURFACE ( 'NONE', #7518, 1.000000000000000000, 0.5000000000000000000 ) ;
#8320=VECTOR ( 'NONE', #11159, 1000.000000000000000 ) ;
#8322=DIRECTION ( 'NONE',  ( 0.000000000000000000, 1.000000000000000000, 0.000000000000000000 ) ) ;
#8326=VERTEX_POINT ( 'NONE', #13628 ) ;
#8328=VERTEX_POINT ( 'NONE', #11275 ) ;
#8331=EDGE_CURVE ( 'NONE', #5911, #9609, #10021, .T. ) ;
#8334=EDGE_LOOP ( 'NONE', ( #11564, #1972, #14575, #1431 ) ) ;
#8342=DIRECTION ( 'NONE',  ( 0.000000000000000000, 0.000000000000000000, -1.000000000000000000 ) ) ;
#8343=CARTESIAN_POINT ( 'NONE',  ( 190.5000000000000568, -179.8058001507315566, -51.45141194869120227 ) ) ;
#8345=VERTEX_POINT ( 'NONE', #6550 ) ;
#8346=EDGE_CURVE ( 'NONE', #13140, #5990, #12448, .T. ) ;
#8347=CIRCLE ( 'NONE', #1518, 0.5000000000000004441 ) ;
#8351=DIRECTION ( 'NONE',  ( 0.000000000000000000, 0.1391731009600592484, 0.9902680687415712502 ) ) ;
#8352=LINE ( 'NONE', #6047, #618 ) ;
#8363=EDGE_CURVE ( 'NONE', #7029, #3604, #14568, .T. ) ;
#8364=DIRECTION ( 'NONE',  ( 0.000000000000000000, -0.1391731009600592484, 0.9902680687415712502 ) ) ;
#8365=DIRECTION ( 'NONE',  ( -0.000000000000000000, 1.000000000000000000, 0.000000000000000000 ) ) ;
#8370=DIRECTION ( 'NONE',  ( 1.000000000000000000, -2.751328491981765035E-32, 3.965082230804130220E-16 ) ) ;
#8373=CIRCLE ( 'NONE', #3066, 1.500000000000001332 ) ;
#8377=DIRECTION ( 'NONE',  ( -0.000000000000000000, -0.9902680687415705840, -0.1391731009600641333 ) ) ;
#8378=DIRECTION ( 'NONE',  ( 0.000000000000000000, 0.9902680687415710281, -0.1391731009600611635 ) ) ;
#8379=DIRECTION ( 'NONE',  ( -1.000000000000000000, 0.000000000000000000, 0.000000000000000000 ) ) ;
#8381=DIRECTION ( 'NONE',  ( 1.000000000000000000, 2.751328491981765035E-32, -3.965082230804130220E-16 ) ) ;
#8383=ADVANCED_FACE ( 'NONE', ( #11126 ), #10172, .T. ) ;
#8390=ORIENTED_EDGE ( 'NONE', *, *, #5973, .T. ) ;
#8394=CARTESIAN_POINT ( 'NONE',  ( -61.94838851346079167, -178.8058001507315566, 52.19066787724494816 ) ) ;
#8397=VECTOR ( 'NONE', #3125, 1000.000000000000000 ) ;
#8400=ORIENTED_EDGE ( 'NONE', *, *, #14212, .F. ) ;
#8405=DIRECTION ( 'NONE',  ( 0.000000000000000000, 0.000000000000000000, -1.000000000000000000 ) ) ;
#8409=ORIENTED_EDGE ( 'NONE', *, *, #10450, .T. ) ;
#8412=EDGE_CURVE ( 'NONE', #176, #12405, #1221, .T. ) ;
#8414=CARTESIAN_POINT ( 'NONE',  ( -70.00000000000000000, 17.53993994372673626, 45.99999999999998579 ) ) ;
#8416=ORIENTED_EDGE ( 'NONE', *, *, #7764, .F. ) ;
#8429=ORIENTED_EDGE ( 'NONE', *, *, #10376, .T. ) ;
#8432=VECTOR ( 'NONE', #3940, 1000.000000000000000 ) ;
#8435=ORIENTED_EDGE ( 'NONE', *, *, #4535, .F. ) ;
#8442=DIRECTION ( 'NONE',  ( 0.000000000000000000, 0.000000000000000000, 1.000000000000000000 ) ) ;
#8443=FACE_OUTER_BOUND ( 'NONE', #888, .T. ) ;
#8454=AXIS2_PLACEMENT_3D ( 'NONE', #14031, #15280, #12998 ) ;
#8455=EDGE_LOOP ( 'NONE', ( #4280, #13616, #3557, #2308 ) ) ;
#8457=CARTESIAN_POINT ( 'NONE',  ( 190.5000000000000853, -179.3753867012116530, 64.38864891670806401 ) ) ;
#8458=CARTESIAN_POINT ( 'NONE',  ( 190.5000000000000568, 16.03993994372673981, -17.50000000000002487 ) ) ;
#8464=EDGE_LOOP ( 'NONE', ( #12971, #13433, #3574, #6175 ) ) ;
#8467=CARTESIAN_POINT ( 'NONE',  ( 190.0000000000000568, 15.03993994372673981, -3.075184203610571654 ) ) ;
#8474=AXIS2_PLACEMENT_3D ( 'NONE', #2313, #14223, #14455 ) ;
#8476=DIRECTION ( 'NONE',  ( 0.000000000000000000, 0.000000000000000000, -1.000000000000000000 ) ) ;
#8483=EDGE_CURVE ( 'NONE', #2454, #552, #1864, .T. ) ;
#8484=ORIENTED_EDGE ( 'NONE', *, *, #6451, .T. ) ;
#8486=CARTESIAN_POINT ( 'NONE',  ( 114.0000000000000426, 15.03993994372673981, 10.05257423913146475 ) ) ;
#8493=EDGE_LOOP ( 'NONE', ( #6487, #12168 ) ) ;
#8497=CYLINDRICAL_SURFACE ( 'NONE', #11090, 0.4999999999999996114 ) ;
#8503=CARTESIAN_POINT ( 'NONE',  ( -76.00000000000001421, -178.8753867012115961, -29.82329228561640022 ) ) ;
#8505=DIRECTION ( 'NONE',  ( 0.000000000000000000, 0.000000000000000000, 1.000000000000000000 ) ) ;
#8506=ORIENTED_EDGE ( 'NONE', *, *, #10393, .T. ) ;
#8508=DIRECTION ( 'NONE',  ( 0.000000000000000000, 0.9902680687415712502, 0.1391731009600584990 ) ) ;
#8513=DIRECTION ( 'NONE',  ( 1.000000000000000000, -0.000000000000000000, -0.000000000000000000 ) ) ;
#8515=ADVANCED_FACE ( 'NONE', ( #987 ), #15198, .T. ) ;
#8520=FACE_OUTER_BOUND ( 'NONE', #148, .T. ) ;
#8521=ORIENTED_EDGE ( 'NONE', *, *, #10550, .T. ) ;
#8527=DIRECTION ( 'NONE',  ( 0.000000000000000000, 0.000000000000000000, -1.000000000000000000 ) ) ;
#8533=CIRCLE ( 'NONE', #11292, 0.5000000000000004441 ) ;
#8534=EDGE_CURVE ( 'NONE', #12812, #1838, #6579, .T. ) ;
#8535=VECTOR ( 'NONE', #14089, 1000.000000000000000 ) ;
#8537=DIRECTION ( 'NONE',  ( 0.000000000000000000, -5.551115123125777653E-14, -1.000000000000000000 ) ) ;
#8538=EDGE_LOOP ( 'NONE', ( #4963, #12010, #7250, #4452 ) ) ;
#8540=ORIENTED_EDGE ( 'NONE', *, *, #6824, .T. ) ;
#8541=DIRECTION ( 'NONE',  ( 1.000000000000000000, 0.000000000000000000, 0.000000000000000000 ) ) ;
#8544=AXIS2_PLACEMENT_3D ( 'NONE', #9108, #5774, #4588 ) ;
#8547=AXIS2_PLACEMENT_3D ( 'NONE', #13050, #10708, #5810 ) ;
#8548=EDGE_CURVE ( 'NONE', #12308, #2407, #9586, .T. ) ;
#8554=ORIENTED_EDGE ( 'NONE', *, *, #11926, .T. ) ;
#8559=ORIENTED_EDGE ( 'NONE', *, *, #9842, .F. ) ;
#8563=ADVANCED_FACE ( 'NONE', ( #2105 ), #6938, .F. ) ;
#8564=PLANE ( 'NONE',  #14835 ) ;
#8566=EDGE_CURVE ( 'NONE', #1955, #1358, #1766, .T. ) ;
#8570=VECTOR ( 'NONE', #13664, 1000.000000000000000 ) ;
#8575=ORIENTED_EDGE ( 'NONE', *, *, #1310, .T. ) ;
#8577=CARTESIAN_POINT ( 'NONE',  ( -63.50000000000002842, 16.03993994372673981, 10.05257423913146475 ) ) ;
#8580=AXIS2_PLACEMENT_3D ( 'NONE', #3178, #2363, #796 ) ;
#8586=VERTEX_POINT ( 'NONE', #14324 ) ;
#8588=CARTESIAN_POINT ( 'NONE',  ( 190.5000000000000853, 16.03993994372673626, 52.49999999999997868 ) ) ;
#8590=FACE_BOUND ( 'NONE', #12424, .T. ) ;
#8595=FACE_OUTER_BOUND ( 'NONE', #2980, .T. ) ;
#8597=DIRECTION ( 'NONE',  ( 0.000000000000000000, -0.9902680687415712502, -0.1391731009600584990 ) ) ;
#8601=ORIENTED_EDGE ( 'NONE', *, *, #335, .F. ) ;
#8605=DIRECTION ( 'NONE',  ( 0.000000000000000000, -4.956352788505162775E-17, 1.000000000000000000 ) ) ;
#8607=DIRECTION ( 'NONE',  ( -1.000000000000000000, -0.000000000000000000, 0.000000000000000000 ) ) ;
#8613=EDGE_CURVE ( 'NONE', #2939, #1838, #13219, .T. ) ;
#8615=ORIENTED_EDGE ( 'NONE', *, *, #10464, .F. ) ;
#8617=ORIENTED_EDGE ( 'NONE', *, *, #9049, .F. ) ;
#8621=ORIENTED_EDGE ( 'NONE', *, *, #3920, .F. ) ;
#8622=DIRECTION ( 'NONE',  ( 1.000000000000000000, 0.000000000000000000, 0.000000000000000000 ) ) ;
#8624=EDGE_CURVE ( 'NONE', #8197, #8640, #11603, .T. ) ;
#8627=AXIS2_PLACEMENT_3D ( 'NONE', #9287, #14084, #3285 ) ;
#8628=ORIENTED_EDGE ( 'NONE', *, *, #7640, .F. ) ;
#8631=DIRECTION ( 'NONE',  ( -1.000000000000000000, 0.000000000000000000, 0.000000000000000000 ) ) ;
#8640=VERTEX_POINT ( 'NONE', #3523 ) ;
#8641=COLOUR_RGB ( '', 0.40784314, 0.44705882, 0.49803922) ;
#8643=CARTESIAN_POINT ( 'NONE',  ( -76.00000000000001421, -178.8058001507315566, -30.31842631998718574 ) ) ;
#8645=AXIS2_PLACEMENT_3D ( 'NONE', #1323, #8379, #13317 ) ;
#8646=CARTESIAN_POINT ( 'NONE',  ( -63.50000000000002842, 15.53993994372673981, -3.075184203610571654 ) ) ;
#8648=SHAPE_REPRESENTATION ( 'Cast Iron Frame Side Blocks x2', ( #12337 ), #180 ) ;
#8652=DIRECTION ( 'NONE',  ( 0.000000000000000000, 1.000000000000000000, 6.938893903907227145E-17 ) ) ;
#8653=LINE ( 'NONE', #3186, #2403 ) ;
#8657=EDGE_CURVE ( 'NONE', #15235, #6079, #14555, .T. ) ;
#8662=ORIENTED_EDGE ( 'NONE', *, *, #5038, .F. ) ;
#8664=EDGE_CURVE ( 'NONE', #14199, #9410, #14371, .T. ) ;
#8665=VECTOR ( 'NONE', #6233, 1000.000000000000000 ) ;
#8666=CARTESIAN_POINT ( 'NONE',  ( 175.9483885134608272, -179.3058001507315566, 52.76585208085545275 ) ) ;
#8670=CARTESIAN_POINT ( 'NONE',  ( 178.0000000000000853, 15.53993994372673981, -17.50000000000002487 ) ) ;
#8671=EDGE_CURVE ( 'NONE', #830, #9239, #9690, .T. ) ;
#8678=DIRECTION ( 'NONE',  ( 0.000000000000000000, 0.000000000000000000, -1.000000000000000000 ) ) ;
#8686=CARTESIAN_POINT ( 'NONE',  ( 177.5000000000000853, -179.8058001507315566, -30.31842631998718574 ) ) ;
#8693=CARTESIAN_POINT ( 'NONE',  ( -76.00000000000001421, 16.03993994372673981, -17.50000000000002487 ) ) ;
#8697=VERTEX_POINT ( 'NONE', #1597 ) ;
#8704=CYLINDRICAL_SURFACE ( 'NONE', #5107, 0.5000000000000000000 ) ;
#8713=DIRECTION ( 'NONE',  ( 0.000000000000000000, 1.000000000000000000, 0.000000000000000000 ) ) ;
#8714=EDGE_LOOP ( 'NONE', ( #5489, #3676, #8957, #612 ) ) ;
#8715=ORIENTED_EDGE ( 'NONE', *, *, #436, .T. ) ;
#8716=LINE ( 'NONE', #7533, #2741 ) ;
#8719=DIRECTION ( 'NONE',  ( -3.965082230804130220E-16, 1.090924371466202084E-47, 1.000000000000000000 ) ) ;
#8724=DIRECTION ( 'NONE',  ( -0.000000000000000000, -0.9902680687415712502, -0.1391731009600586100 ) ) ;
#8726=ORIENTED_EDGE ( 'NONE', *, *, #2736, .T. ) ;
#8727=DIRECTION ( 'NONE',  ( 1.000000000000000000, -0.000000000000000000, -0.000000000000000000 ) ) ;
#8734=ORIENTED_EDGE ( 'NONE', *, *, #1797, .F. ) ;
#8742=CARTESIAN_POINT ( 'NONE',  ( 178.0000000000000853, -179.8058001507315566, 52.49999999999997868 ) ) ;
#8747=LINE ( 'NONE', #3689, #10397 ) ;
#8748=EDGE_LOOP ( 'NONE', ( #14383, #9016, #739, #7604 ) ) ;
#8749=DIRECTION ( 'NONE',  ( 0.000000000000000000, 4.956352788505162775E-17, -1.000000000000000000 ) ) ;
#8750=ORIENTED_EDGE ( 'NONE', *, *, #731, .T. ) ;
#8754=DIRECTION ( 'NONE',  ( 5.518327896226364679E-17, -0.9902680687415713612, 0.1391731009600582492 ) ) ;
#8759=ADVANCED_FACE ( 'NONE', ( #11633 ), #4029, .T. ) ;
#8761=EDGE_CURVE ( 'NONE', #10463, #14752, #13884, .T. ) ;
#8765=ORIENTED_EDGE ( 'NONE', *, *, #10324, .F. ) ;
#8770=ADVANCED_FACE ( 'NONE', ( #10336 ), #13875, .T. ) ;
#8771=VERTEX_POINT ( 'NONE', #12689 ) ;
#8774=CIRCLE ( 'NONE', #2221, 0.4999999999999998890 ) ;
#8775=CARTESIAN_POINT ( 'NONE',  ( 184.0000000000000568, 17.53993994372673981, -12.49999999999999289 ) ) ;
#8776=ORIENTED_EDGE ( 'NONE', *, *, #14212, .T. ) ;
#8777=AXIS2_PLACEMENT_3D ( 'NONE', #1819, #6662, #8867 ) ;
#8782=ORIENTED_EDGE ( 'NONE', *, *, #13150, .T. ) ;
#8783=FACE_BOUND ( 'NONE', #6391, .T. ) ;
#8784=CIRCLE ( 'NONE', #1963, 0.4999999999999998890 ) ;
#8785=EDGE_CURVE ( 'NONE', #9678, #13452, #9234, .T. ) ;
#8788=ORIENTED_EDGE ( 'NONE', *, *, #3081, .F. ) ;
#8792=CIRCLE ( 'NONE', #14562, 0.5000000000000004441 ) ;
#8794=VERTEX_POINT ( 'NONE', #5445 ) ;
#8799=AXIS2_PLACEMENT_3D ( 'NONE', #9456, #9379, #2182 ) ;
#8802=AXIS2_PLACEMENT_3D ( 'NONE', #3671, #9845, #9919 ) ;
#8807=LINE ( 'NONE', #1841, #10567 ) ;
#8808=VERTEX_POINT ( 'NONE', #1950 ) ;
#8818=MECHANICAL_DESIGN_GEOMETRIC_PRESENTATION_REPRESENTATION('',(#5355),#14346);
#8819=LINE ( 'NONE', #11263, #78 ) ;
#8827=DIRECTION ( 'NONE',  ( -3.862829527358613429E-15, -0.9902680687415705840, 0.1391731009600641333 ) ) ;
#8834=AXIS2_PLACEMENT_3D ( 'NONE', #1149, #13296, #7252 ) ;
#8835=DIRECTION ( 'NONE',  ( -0.000000000000000000, 1.000000000000000000, -0.000000000000000000 ) ) ;
#8839=LINE ( 'NONE', #12760, #3274 ) ;
#8841=ORIENTED_EDGE ( 'NONE', *, *, #9721, .T. ) ;
#8843=AXIS2_PLACEMENT_3D ( 'NONE', #4744, #8322, #13339 ) ;
#8844=CIRCLE ( 'NONE', #10864, 1.000000000000000888 ) ;
#8848=EDGE_LOOP ( 'NONE', ( #8416, #1297, #9817, #7814, #1969 ) ) ;
#8849=ADVANCED_FACE ( 'NONE', ( #13963 ), #4563, .T. ) ;
#8851=EDGE_CURVE ( 'NONE', #9167, #2929, #12767, .T. ) ;
#8852=EDGE_CURVE ( 'NONE', #12081, #620, #8347, .T. ) ;
#8857=CARTESIAN_POINT ( 'NONE',  ( -63.50000000000002842, 15.53993994372673981, -17.50000000000002487 ) ) ;
#8858=CYLINDRICAL_SURFACE ( 'NONE', #7599, 0.4999999999999996114 ) ;
#8861=TOROIDAL_SURFACE ( 'NONE', #12877, 1.000000000000000000, 0.5000000000000000000 ) ;
#8867=DIRECTION ( 'NONE',  ( 0.000000000000000000, 0.000000000000000000, -1.000000000000000000 ) ) ;
#8869=DIRECTION ( 'NONE',  ( 0.000000000000000000, -0.9902680687415713612, 0.1391731009600582492 ) ) ;
#8874=EDGE_LOOP ( 'NONE', ( #8782, #15539, #11389, #2632 ) ) ;
#8877=VERTEX_POINT ( 'NONE', #13306 ) ;
#8889=ORIENTED_EDGE ( 'NONE', *, *, #8657, .F. ) ;
#8893=DIRECTION ( 'NONE',  ( 1.000000000000000000, -2.751328491981765035E-32, 3.965082230804130220E-16 ) ) ;
#8900=DIRECTION ( 'NONE',  ( -3.965082230804130220E-16, 0.000000000000000000, 1.000000000000000000 ) ) ;
#8904=DIRECTION ( 'NONE',  ( 0.000000000000000000, -0.1391731009600586100, 0.9902680687415712502 ) ) ;
#8906=ORIENTED_EDGE ( 'NONE', *, *, #12884, .T. ) ;
#8908=DIRECTION ( 'NONE',  ( 0.000000000000000000, 0.000000000000000000, 1.000000000000000000 ) ) ;
#8911=AXIS2_PLACEMENT_3D ( 'NONE', #10918, #11146, #7441 ) ;
#8912=DIRECTION ( 'NONE',  ( 0.000000000000000000, -0.000000000000000000, -1.000000000000000000 ) ) ;
#8921=AXIS2_PLACEMENT_3D ( 'NONE', #1871, #15357, #5675 ) ;
#8922=ORIENTED_EDGE ( 'NONE', *, *, #11197, .F. ) ;
#8924=VECTOR ( 'NONE', #7096, 1000.000000000000000 ) ;
#8938=CARTESIAN_POINT ( 'NONE',  ( -64.00000000000002842, -179.8058001507315566, 84.88378295107887084 ) ) ;
#8940=FACE_OUTER_BOUND ( 'NONE', #6105, .T. ) ;
#8941=ORIENTED_EDGE ( 'NONE', *, *, #10592, .T. ) ;
#8942=VECTOR ( 'NONE', #10891, 1000.000000000000000 ) ;
#8943=ADVANCED_FACE ( 'NONE', ( #4844 ), #5787, .T. ) ;
#8945=ORIENTED_EDGE ( 'NONE', *, *, #13409, .T. ) ;
#8946=AXIS2_PLACEMENT_3D ( 'NONE', #14982, #7678, #5532 ) ;
#8947=EDGE_CURVE ( 'NONE', #815, #12968, #7336, .T. ) ;
#8950=CARTESIAN_POINT ( 'NONE',  ( 190.0000000000000568, -179.3058001507315566, -51.45141194869120227 ) ) ;
#8951=CARTESIAN_POINT ( 'NONE',  ( 190.0000000000000568, -178.8058001507315566, -30.31842631998718574 ) ) ;
#8954=CARTESIAN_POINT ( 'NONE',  ( -64.00000000000002842, -178.8058001507315566, -30.31842631998718574 ) ) ;
#8956=CIRCLE ( 'NONE', #2128, 0.5000000000000001110 ) ;
#8957=ORIENTED_EDGE ( 'NONE', *, *, #15518, .T. ) ;
#8961=LINE ( 'NONE', #11397, #12739 ) ;
#8965=VECTOR ( 'NONE', #4938, 1000.000000000000000 ) ;
#8967=ORIENTED_EDGE ( 'NONE', *, *, #9496, .T. ) ;
#8971=FACE_OUTER_BOUND ( 'NONE', #201, .T. ) ;
#8976=EDGE_CURVE ( 'NONE', #12405, #15483, #4603, .T. ) ;
#8980=VECTOR ( 'NONE', #3738, 1000.000000000000000 ) ;
#8983=ORIENTED_EDGE ( 'NONE', *, *, #4111, .T. ) ;
#8984=DIRECTION ( 'NONE',  ( -1.000000000000000000, 0.000000000000000000, 0.000000000000000000 ) ) ;
#8985=AXIS2_PLACEMENT_3D ( 'NONE', #8053, #838, #9306 ) ;
#8987=DIRECTION ( 'NONE',  ( 1.000000000000000000, -0.000000000000000000, -0.000000000000000000 ) ) ;
#8988=ORIENTED_EDGE ( 'NONE', *, *, #2766, .T. ) ;
#8990=CARTESIAN_POINT ( 'NONE',  ( -64.00000000000002842, -178.9449732516916072, 64.32815825124539799 ) ) ;
#8992=ADVANCED_FACE ( 'NONE', ( #13189 ), #1190, .F. ) ;
#9001=DIRECTION ( 'NONE',  ( 0.000000000000000000, 1.000000000000000000, 6.938893903907227145E-17 ) ) ;
#9003=LINE ( 'NONE', #9879, #4071 ) ;
#9009=AXIS2_PLACEMENT_3D ( 'NONE', #14808, #3934, #1475 ) ;
#9011=ORIENTED_EDGE ( 'NONE', *, *, #4093, .F. ) ;
#9012=CARTESIAN_POINT ( 'NONE',  ( -76.50000000000002842, -178.8058001507315566, 53.19066787724494816 ) ) ;
#9016=ORIENTED_EDGE ( 'NONE', *, *, #989, .T. ) ;
#9022=ORIENTED_EDGE ( 'NONE', *, *, #7503, .T. ) ;
#9033=AXIS2_PLACEMENT_3D ( 'NONE', #15440, #13153, #3095 ) ;
#9034=CARTESIAN_POINT ( 'NONE',  ( 178.0000000000000853, -179.8058001507315566, 65.31842631998698323 ) ) ;
#9039=VERTEX_POINT ( 'NONE', #2153 ) ;
#9043=FACE_OUTER_BOUND ( 'NONE', #6090, .T. ) ;
#9049=EDGE_CURVE ( 'NONE', #9280, #5867, #13031, .T. ) ;
#9051=CIRCLE ( 'NONE', #14321, 0.5000000000000001110 ) ;
#9052=LINE ( 'NONE', #14867, #12697 ) ;
#9055=DIRECTION ( 'NONE',  ( -1.000000000000000000, -2.751328491981765035E-32, 3.965082230804130220E-16 ) ) ;
#9057=ORIENTED_EDGE ( 'NONE', *, *, #10464, .T. ) ;
#9058=CARTESIAN_POINT ( 'NONE',  ( 184.0000000000000568, 17.53993994372673626, 47.49999999999997868 ) ) ;
#9060=DIRECTION ( 'NONE',  ( -9.657073818396194363E-16, -0.9902680687415711391, 0.1391731009600592484 ) ) ;
#9065=DIRECTION ( 'NONE',  ( -1.000000000000000000, 0.000000000000000000, 0.000000000000000000 ) ) ;
#9066=AXIS2_PLACEMENT_3D ( 'NONE', #10526, #1124, #2233 ) ;
#9067=EDGE_LOOP ( 'NONE', ( #9151, #4759, #1278, #450 ) ) ;
#9070=CARTESIAN_POINT ( 'NONE',  ( -61.94838851346079167, -179.3058001507315566, 84.88378295107887084 ) ) ;
#9073=DIRECTION ( 'NONE',  ( 0.000000000000000000, 0.000000000000000000, -1.000000000000000000 ) ) ;
#9075=DIRECTION ( 'NONE',  ( 3.965082230804130220E-16, -0.000000000000000000, -1.000000000000000000 ) ) ;
#9076=CIRCLE ( 'NONE', #6296, 1.500000000000001332 ) ;
#9078=CARTESIAN_POINT ( 'NONE',  ( -64.00000000000002842, 15.53993994372673804, 38.07518420361041933 ) ) ;
#9079=DIRECTION ( 'NONE',  ( 0.000000000000000000, -1.000000000000000000, -6.938893903907222067E-15 ) ) ;
#9085=AXIS2_PLACEMENT_3D ( 'NONE', #10847, #14067, #3262 ) ;
#9086=AXIS2_PLACEMENT_3D ( 'NONE', #5998, #7861, #4356 ) ;
#9088=CARTESIAN_POINT ( 'NONE',  ( 0.000000000000000000, 15.53993994372673981, 7.305634244248866343E-16 ) ) ;
#9090=CIRCLE ( 'NONE', #3034, 0.5000000000000001110 ) ;
#9092=PLANE ( 'NONE',  #11208 ) ;
#9093=DIRECTION ( 'NONE',  ( 1.000000000000000000, -0.000000000000000000, -0.000000000000000000 ) ) ;
#9094=CIRCLE ( 'NONE', #12600, 0.5000000000000001110 ) ;
#9095=CYLINDRICAL_SURFACE ( 'NONE', #9922, 0.5000000000000004441 ) ;
#9097=AXIS2_PLACEMENT_3D ( 'NONE', #3296, #14096, #5816 ) ;
#9108=CARTESIAN_POINT ( 'NONE',  ( 184.0000000000000568, 15.53993994372673626, 47.49999999999997868 ) ) ;
#9111=AXIS2_PLACEMENT_3D ( 'NONE', #6627, #7811, #1632 ) ;
#9112=EDGE_LOOP ( 'NONE', ( #1376, #6772, #1279, #14947 ) ) ;
#9116=CARTESIAN_POINT ( 'NONE',  ( -70.00000000000000000, -201.3058001507315566, 76.45141194869098911 ) ) ;
#9117=DIRECTION ( 'NONE',  ( 1.000000000000000000, -0.000000000000000000, -0.000000000000000000 ) ) ;
#9118=VECTOR ( 'NONE', #8245, 1000.000000000000000 ) ;
#9121=TOROIDAL_SURFACE ( 'NONE', #9378, 1.000000000000000000, 0.5000000000000000000 ) ;
#9123=CARTESIAN_POINT ( 'NONE',  ( 190.0000000000000568, 15.53993994372673981, -3.075184203610571654 ) ) ;
#9125=CARTESIAN_POINT ( 'NONE',  ( 190.0000000000001137, -178.8058001507315566, 65.31842631998698323 ) ) ;
#9133=CARTESIAN_POINT ( 'NONE',  ( 190.5000000000000853, 17.53993994372673626, 52.49999999999997868 ) ) ;
#9135=DIRECTION ( 'NONE',  ( 0.000000000000000000, 0.1391731009600592484, 0.9902680687415712502 ) ) ;
#9138=ADVANCED_FACE ( 'NONE', ( #10594 ), #15463, .F. ) ;
#9151=ORIENTED_EDGE ( 'NONE', *, *, #11407, .F. ) ;
#9152=DIRECTION ( 'NONE',  ( 0.000000000000000000, 0.000000000000000000, -1.000000000000000000 ) ) ;
#9155=DIRECTION ( 'NONE',  ( 1.000000000000000000, 0.000000000000000000, 0.000000000000000000 ) ) ;
#9160=ADVANCED_FACE ( 'NONE', ( #11038 ), #11703, .T. ) ;
#9161=DIRECTION ( 'NONE',  ( -0.000000000000000000, -0.9902680687415702510, -0.1391731009600660485 ) ) ;
#9167=VERTEX_POINT ( 'NONE', #3327 ) ;
#9170=FACE_OUTER_BOUND ( 'NONE', #332, .T. ) ;
#9179=ORIENTED_EDGE ( 'NONE', *, *, #15518, .F. ) ;
#9190=DIRECTION ( 'NONE',  ( 1.000000000000000000, -2.751328491981765035E-32, 3.965082230804130220E-16 ) ) ;
#9191=EDGE_CURVE ( 'NONE', #12014, #6280, #15377, .T. ) ;
#9194=DIRECTION ( 'NONE',  ( -0.000000000000000000, -0.000000000000000000, -1.000000000000000000 ) ) ;
#9195=DIRECTION ( 'NONE',  ( 0.000000000000000000, 0.000000000000000000, 1.000000000000000000 ) ) ;
#9197=CYLINDRICAL_SURFACE ( 'NONE', #10585, 0.5000000000000004441 ) ;
#9202=DIRECTION ( 'NONE',  ( -0.000000000000000000, 1.000000000000000000, 6.938893903907227145E-17 ) ) ;
#9208=LINE ( 'NONE', #15027, #377 ) ;
#9212=DIRECTION ( 'NONE',  ( 0.000000000000000000, 6.938893903907227145E-17, -1.000000000000000000 ) ) ;
#9214=CARTESIAN_POINT ( 'NONE',  ( 178.0000000000000853, 23.05038067821381986, -0.9395626039331514967 ) ) ;
#9220=AXIS2_PLACEMENT_3D ( 'NONE', #9447, #12981, #7319 ) ;
#9229=DIRECTION ( 'NONE',  ( 0.000000000000000000, 0.000000000000000000, -1.000000000000000000 ) ) ;
#9234=LINE ( 'NONE', #6949, #238 ) ;
#9239=VERTEX_POINT ( 'NONE', #4079 ) ;
#9241=LINE ( 'NONE', #13803, #4575 ) ;
#9247=CIRCLE ( 'NONE', #904, 0.5000000000000004441 ) ;
#9249=DIRECTION ( 'NONE',  ( 0.000000000000000000, 0.000000000000000000, -1.000000000000000000 ) ) ;
#9256=ORIENTED_EDGE ( 'NONE', *, *, #2314, .T. ) ;
#9257=VECTOR ( 'NONE', #12376, 1000.000000000000000 ) ;
#9259=ADVANCED_FACE ( 'NONE', ( #7732 ), #2672, .T. ) ;
#9260=CARTESIAN_POINT ( 'NONE',  ( -61.94838851346079167, -179.3058001507315566, -29.88378295107906624 ) ) ;
#9261=VERTEX_POINT ( 'NONE', #5114 ) ;
#9263=LINE ( 'NONE', #6896, #4743 ) ;
#9264=CARTESIAN_POINT ( 'NONE',  ( -70.00000000000000000, 15.53993994372673981, -10.99999999999999645 ) ) ;
#9266=CARTESIAN_POINT ( 'NONE',  ( -70.00000000000000000, -179.3058001507315566, 74.95141194869098911 ) ) ;
#9268=FACE_OUTER_BOUND ( 'NONE', #3594, .T. ) ;
#9272=EDGE_CURVE ( 'NONE', #13191, #4430, #12597, .T. ) ;
#9276=DIRECTION ( 'NONE',  ( 0.000000000000000000, 0.000000000000000000, 1.000000000000000000 ) ) ;
#9277=EDGE_LOOP ( 'NONE', ( #698, #15389, #4129, #5975 ) ) ;
#9280=VERTEX_POINT ( 'NONE', #11345 ) ;
#9281=LINE ( 'NONE', #11726, #10579 ) ;
#9284=TOROIDAL_SURFACE ( 'NONE', #12542, 1.000000000000000000, 0.5000000000000000000 ) ;
#9287=CARTESIAN_POINT ( 'NONE',  ( -76.00000000000001421, 13.40307322461932493, -2.295403246091865412 ) ) ;
#9289=CARTESIAN_POINT ( 'NONE',  ( 178.0000000000000853, 15.03993994372673804, 38.07518420361041933 ) ) ;
#9295=CARTESIAN_POINT ( 'NONE',  ( 190.0000000000000568, 15.03993994372673804, 24.94742576086838781 ) ) ;
#9302=EDGE_CURVE ( 'NONE', #13002, #11614, #590, .T. ) ;
#9304=FACE_OUTER_BOUND ( 'NONE', #1915, .T. ) ;
#9306=DIRECTION ( 'NONE',  ( 0.000000000000000000, 0.000000000000000000, -1.000000000000000000 ) ) ;
#9317=DIRECTION ( 'NONE',  ( 0.000000000000000000, 0.9902680687415713612, -0.1391731009600582492 ) ) ;
#9318=CARTESIAN_POINT ( 'NONE',  ( -70.00000000000000000, -181.3058001507315566, 77.95141194869098911 ) ) ;
#9320=AXIS2_PLACEMENT_3D ( 'NONE', #14234, #11567, #8193 ) ;
#9322=DIRECTION ( 'NONE',  ( -0.000000000000000000, -0.000000000000000000, 1.000000000000000000 ) ) ;
#9325=CARTESIAN_POINT ( 'NONE',  ( -63.50000000000002842, 17.53993994372673626, 52.49999999999997868 ) ) ;
#9327=TOROIDAL_SURFACE ( 'NONE', #7830, 1.000000000000000000, 0.5000000000000000000 ) ;
#9332=EDGE_CURVE ( 'NONE', #6993, #12750, #247, .T. ) ;
#9334=ORIENTED_EDGE ( 'NONE', *, *, #14428, .F. ) ;
#9337=CARTESIAN_POINT ( 'NONE',  ( -70.00000000000000000, -179.3058001507315566, -39.95141194869120937 ) ) ;
#9338=EDGE_LOOP ( 'NONE', ( #8258, #14571, #424, #6729 ) ) ;
#9339=EDGE_CURVE ( 'NONE', #6971, #2984, #6831, .T. ) ;
#9341=CARTESIAN_POINT ( 'NONE',  ( -76.00000000000004263, 15.17911304468679745, 25.93769382960994818 ) ) ;
#9342=CARTESIAN_POINT ( 'NONE',  ( 175.9483885134608272, -178.8058001507315566, 65.31842631998698323 ) ) ;
#9344=DIRECTION ( 'NONE',  ( -3.965082230804130220E-16, 4.956352788505162775E-17, -1.000000000000000000 ) ) ;
#9345=CARTESIAN_POINT ( 'NONE',  ( -76.00000000000001421, 14.90076684276668040, -2.084916134869001958 ) ) ;
#9346=VECTOR ( 'NONE', #4786, 1000.000000000000000 ) ;
#9350=ORIENTED_EDGE ( 'NONE', *, *, #6508, .F. ) ;
#9353=DIRECTION ( 'NONE',  ( -0.000000000000000000, 1.000000000000000000, -0.000000000000000000 ) ) ;
#9354=EDGE_LOOP ( 'NONE', ( #15477, #7724, #10924, #14866 ) ) ;
#9357=ADVANCED_FACE ( 'NONE', ( #13471 ), #1465, .T. ) ;
#9358=ORIENTED_EDGE ( 'NONE', *, *, #4596, .T. ) ;
#9360=FACE_OUTER_BOUND ( 'NONE', #12386, .T. ) ;
#9361=AXIS2_PLACEMENT_3D ( 'NONE', #48, #4885, #14495 ) ;
#9367=CARTESIAN_POINT ( 'NONE',  ( 190.0000000000000853, -178.7362136002515172, 52.68580191161573367 ) ) ;
#9369=EDGE_LOOP ( 'NONE', ( #13626, #10744, #239, #8506 ) ) ;
#9370=DIRECTION ( 'NONE',  ( 1.000000000000000000, 0.000000000000000000, 0.000000000000000000 ) ) ;
#9374=AXIS2_PLACEMENT_3D ( 'NONE', #10577, #4722, #8151 ) ;
#9378=AXIS2_PLACEMENT_3D ( 'NONE', #10945, #1293, #12188 ) ;
#9379=DIRECTION ( 'NONE',  ( -0.000000000000000000, 1.000000000000000000, -0.000000000000000000 ) ) ;
#9380=DIRECTION ( 'NONE',  ( -1.000000000000000000, 0.000000000000000000, 0.000000000000000000 ) ) ;
#9386=VECTOR ( 'NONE', #9403, 1000.000000000000000 ) ;
#9388=FACE_OUTER_BOUND ( 'NONE', #11380, .T. ) ;
#9390=ORIENTED_EDGE ( 'NONE', *, *, #8098, .T. ) ;
#9391=ORIENTED_EDGE ( 'NONE', *, *, #14681, .T. ) ;
#9392=DIRECTION ( 'NONE',  ( 1.000000000000000000, 0.000000000000000000, 0.000000000000000000 ) ) ;
#9403=DIRECTION ( 'NONE',  ( -1.000000000000000000, -0.000000000000000000, -0.000000000000000000 ) ) ;
#9406=DIRECTION ( 'NONE',  ( 1.000000000000000000, 0.000000000000000000, 0.000000000000000000 ) ) ;
#9410=VERTEX_POINT ( 'NONE', #14170 ) ;
#9414=VECTOR ( 'NONE', #5062, 1000.000000000000000 ) ;
#9415=ORIENTED_EDGE ( 'NONE', *, *, #12469, .F. ) ;
#9416=DIRECTION ( 'NONE',  ( 0.000000000000000000, -0.1391731009600591096, 0.9902680687415711391 ) ) ;
#9421=EDGE_CURVE ( 'NONE', #5266, #5077, #8844, .T. ) ;
#9423=DIRECTION ( 'NONE',  ( 1.000000000000000000, -6.938893903907222067E-15, 0.000000000000000000 ) ) ;
#9435=EDGE_CURVE ( 'NONE', #7302, #11235, #14644, .T. ) ;
#9436=AXIS2_PLACEMENT_3D ( 'NONE', #12050, #8513, #2584 ) ;
#9437=FACE_OUTER_BOUND ( 'NONE', #986, .T. ) ;
#9439=ADVANCED_FACE ( 'NONE', ( #8042 ), #10622, .T. ) ;
#9446=VERTEX_POINT ( 'NONE', #4547 ) ;
#9447=CARTESIAN_POINT ( 'NONE',  ( 190.5000000000000853, 15.03993994372673804, 24.94742576086838781 ) ) ;
#9452=DIRECTION ( 'NONE',  ( 0.000000000000000000, -0.1391731009600591096, 0.9902680687415711391 ) ) ;
#9454=ORIENTED_EDGE ( 'NONE', *, *, #11053, .T. ) ;
#9456=CARTESIAN_POINT ( 'NONE',  ( -70.00000000000000000, -181.3058001507315566, -41.45141194869120227 ) ) ;
#9458=AXIS2_PLACEMENT_3D ( 'NONE', #3127, #584, #1931 ) ;
#9460=CARTESIAN_POINT ( 'NONE',  ( -61.94838851346079167, -179.3058001507315566, 52.76585208085545275 ) ) ;
#9464=FACE_OUTER_BOUND ( 'NONE', #10321, .T. ) ;
#9467=EDGE_CURVE ( 'NONE', #14786, #14360, #1860, .T. ) ;
#9471=ORIENTED_EDGE ( 'NONE', *, *, #14042, .F. ) ;
#9472=DIRECTION ( 'NONE',  ( 0.000000000000000000, 0.000000000000000000, 1.000000000000000000 ) ) ;
#9473=DIRECTION ( 'NONE',  ( -1.000000000000000000, -2.751328491981765035E-32, 3.965082230804130220E-16 ) ) ;
#9476=CIRCLE ( 'NONE', #4932, 1.499999999999997780 ) ;
#9479=EDGE_CURVE ( 'NONE', #6496, #8326, #11816, .T. ) ;
#9486=CIRCLE ( 'NONE', #129, 0.5000000000000004441 ) ;
#9489=ORIENTED_EDGE ( 'NONE', *, *, #3840, .F. ) ;
#9490=EDGE_LOOP ( 'NONE', ( #6045, #3370, #6952, #3386 ) ) ;
#9491=DIRECTION ( 'NONE',  ( -0.000000000000000000, -4.956352788505162775E-17, 1.000000000000000000 ) ) ;
#9492=CARTESIAN_POINT ( 'NONE',  ( -70.00000000000000000, 17.53993994372673626, 48.99999999999997158 ) ) ;
#9495=DIRECTION ( 'NONE',  ( -5.518327896226373307E-17, 0.9902680687415712502, 0.1391731009600586100 ) ) ;
#9496=EDGE_CURVE ( 'NONE', #8640, #5077, #746, .T. ) ;
#9513=ORIENTED_EDGE ( 'NONE', *, *, #7777, .T. ) ;
#9521=ADVANCED_FACE ( 'NONE', ( #3519 ), #10875, .T. ) ;
#9528=CARTESIAN_POINT ( 'NONE',  ( -76.50000000000001421, 15.53993994372673804, 38.07518420361041933 ) ) ;
#9529=AXIS2_PLACEMENT_3D ( 'NONE', #4826, #10674, #2534 ) ;
#9530=CARTESIAN_POINT ( 'NONE',  ( -63.50000000000002842, 15.03993994372673804, 38.07518420361041933 ) ) ;
#9533=VECTOR ( 'NONE', #1119, 1000.000000000000000 ) ;
#9536=LINE ( 'NONE', #1157, #11296 ) ;
#9538=AXIS2_PLACEMENT_3D ( 'NONE', #1471, #7493, #12217 ) ;
#9541=CIRCLE ( 'NONE', #5781, 0.5000000000000004441 ) ;
#9542=EDGE_LOOP ( 'NONE', ( #13353, #1965 ) ) ;
#9543=VECTOR ( 'NONE', #6074, 1000.000000000000000 ) ;
#9544=ORIENTED_EDGE ( 'NONE', *, *, #12628, .T. ) ;
#9545=LINE ( 'NONE', #14191, #200 ) ;
#9547=DIRECTION ( 'NONE',  ( 0.000000000000000000, -1.734723475976808672E-15, 1.000000000000000000 ) ) ;
#9548=SURFACE_STYLE_FILL_AREA ( #932 ) ;
#9562=EDGE_LOOP ( 'NONE', ( #11164, #5096, #172, #2696 ) ) ;
#9563=AXIS2_PLACEMENT_3D ( 'NONE', #9088, #10419, #12852 ) ;
#9567=AXIS2_PLACEMENT_3D ( 'NONE', #92, #1132, #9750 ) ;
#9579=DIRECTION ( 'NONE',  ( 0.000000000000000000, 0.000000000000000000, 1.000000000000000000 ) ) ;
#9581=VECTOR ( 'NONE', #4873, 1000.000000000000000 ) ;
#9583=EDGE_LOOP ( 'NONE', ( #10968, #10827, #13172, #12318 ) ) ;
#9586=CIRCLE ( 'NONE', #9097, 0.5000000000000004441 ) ;
#9589=DIRECTION ( 'NONE',  ( 0.000000000000000000, 0.000000000000000000, -1.000000000000000000 ) ) ;
#9590=DIRECTION ( 'NONE',  ( -5.518327896226365911E-17, -0.9902680687415714722, 0.1391731009600582769 ) ) ;
#9593=CIRCLE ( 'NONE', #4536, 0.5000000000000004441 ) ;
#9595=AXIS2_PLACEMENT_3D ( 'NONE', #8211, #12991, #10636 ) ;
#9600=ORIENTED_EDGE ( 'NONE', *, *, #1181, .T. ) ;
#9601=DIRECTION ( 'NONE',  ( 0.000000000000000000, 0.000000000000000000, -1.000000000000000000 ) ) ;
#9605=ORIENTED_EDGE ( 'NONE', *, *, #15503, .T. ) ;
#9609=VERTEX_POINT ( 'NONE', #4869 ) ;
#9611=CARTESIAN_POINT ( 'NONE',  ( -70.00000000000000000, -201.3058001507315566, 74.95141194869098911 ) ) ;
#9615=DIRECTION ( 'NONE',  ( -0.000000000000000000, -0.9902680687415711391, -0.1391731009600592484 ) ) ;
#9616=PLANE ( 'NONE',  #10503 ) ;
#9617=CARTESIAN_POINT ( 'NONE',  ( -63.50000000000002842, -178.9449732516916072, 64.32815825124541220 ) ) ;
#9623=CYLINDRICAL_SURFACE ( 'NONE', #13461, 0.4999999999999996114 ) ;
#9624=DIRECTION ( 'NONE',  ( -0.000000000000000000, -1.000000000000000000, -6.938893903907222067E-15 ) ) ;
#9625=CARTESIAN_POINT ( 'NONE',  ( 190.5000000000000568, -178.8058001507315566, -17.19066787724516843 ) ) ;
#9627=ORIENTED_EDGE ( 'NONE', *, *, #3798, .T. ) ;
#9628=CARTESIAN_POINT ( 'NONE',  ( 178.0000000000000853, 14.97035339324670744, 37.58005016923963382 ) ) ;
#9631=DIRECTION ( 'NONE',  ( 1.000000000000000000, 0.000000000000000000, 0.000000000000000000 ) ) ;
#9633=VECTOR ( 'NONE', #13101, 1000.000000000000000 ) ;
#9638=CIRCLE ( 'NONE', #4841, 0.5000000000000000000 ) ;
#9642=EDGE_LOOP ( 'NONE', ( #2057, #403, #6059, #8788 ) ) ;
#9643=AXIS2_PLACEMENT_3D ( 'NONE', #11659, #5581, #816 ) ;
#9646=ORIENTED_EDGE ( 'NONE', *, *, #364, .F. ) ;
#9647=CARTESIAN_POINT ( 'NONE',  ( 190.5000000000000568, -179.3058001507315566, -51.45141194869120227 ) ) ;
#9648=CIRCLE ( 'NONE', #8645, 0.9999999999999991118 ) ;
#9655=AXIS2_PLACEMENT_3D ( 'NONE', #7601, #10429, #13974 ) ;
#9657=DIRECTION ( 'NONE',  ( -0.000000000000000000, 0.000000000000000000, 1.000000000000000000 ) ) ;
#9661=DIRECTION ( 'NONE',  ( 1.000000000000000000, 2.751328491981765035E-32, -3.965082230804130220E-16 ) ) ;
#9662=EDGE_CURVE ( 'NONE', #14434, #7084, #10371, .T. ) ;
#9669=CIRCLE ( 'NONE', #5124, 0.5000000000000004441 ) ;
#9671=CYLINDRICAL_SURFACE ( 'NONE', #2767, 0.5000000000000004441 ) ;
#9672=CYLINDRICAL_SURFACE ( 'NONE', #2151, 0.4999999999999996114 ) ;
#9673=DIRECTION ( 'NONE',  ( 1.000000000000000000, 2.751328491981765035E-32, -3.965082230804130220E-16 ) ) ;
#9678=VERTEX_POINT ( 'NONE', #13911 ) ;
#9684=ORIENTED_EDGE ( 'NONE', *, *, #11169, .F. ) ;
#9690=LINE ( 'NONE', #14482, #6323 ) ;
#9698=CIRCLE ( 'NONE', #7194, 0.5000000000000001110 ) ;
#9706=AXIS2_PLACEMENT_3D ( 'NONE', #8293, #5184, #3921 ) ;
#9717=AXIS2_PLACEMENT_3D ( 'NONE', #6366, #6444, #14860 ) ;
#9718=ORIENTED_EDGE ( 'NONE', *, *, #13880, .F. ) ;
#9721=EDGE_CURVE ( 'NONE', #7716, #3571, #4307, .T. ) ;
#9722=EDGE_CURVE ( 'NONE', #14048, #12371, #4352, .T. ) ;
#9726=VERTEX_POINT ( 'NONE', #15233 ) ;
#9727=CARTESIAN_POINT ( 'NONE',  ( -61.94838851346079167, -181.3058001507315566, -51.45141194869120227 ) ) ;
#9731=FACE_OUTER_BOUND ( 'NONE', #9939, .T. ) ;
#9733=TOROIDAL_SURFACE ( 'NONE', #2932, 1.000000000000000000, 0.5000000000000000000 ) ;
#9739=CARTESIAN_POINT ( 'NONE',  ( 190.5000000000000853, -179.8058001507315566, 52.19066787724494816 ) ) ;
#9746=ORIENTED_EDGE ( 'NONE', *, *, #10848, .T. ) ;
#9750=DIRECTION ( 'NONE',  ( 0.000000000000000000, 0.000000000000000000, -1.000000000000000000 ) ) ;
#9754=ADVANCED_FACE ( 'NONE', ( #11473 ), #11708, .F. ) ;
#9756=ORIENTED_EDGE ( 'NONE', *, *, #2025, .F. ) ;
#9760=CARTESIAN_POINT ( 'NONE',  ( -76.50000000000001421, 16.03993994372673981, -17.50000000000002487 ) ) ;
#9777=ORIENTED_EDGE ( 'NONE', *, *, #7639, .T. ) ;
#9779=ORIENTED_EDGE ( 'NONE', *, *, #2025, .T. ) ;
#9782=CIRCLE ( 'NONE', #11043, 1.000000000000000888 ) ;
#9788=ORIENTED_EDGE ( 'NONE', *, *, #6508, .T. ) ;
#9789=ADVANCED_FACE ( 'NONE', ( #7769 ), #8861, .T. ) ;
#9791=CIRCLE ( 'NONE', #2987, 0.5000000000000001110 ) ;
#9793=EDGE_LOOP ( 'NONE', ( #12213, #2858, #11954, #4187 ) ) ;
#9797=ORIENTED_EDGE ( 'NONE', *, *, #12260, .F. ) ;
#9800=ORIENTED_EDGE ( 'NONE', *, *, #12306, .F. ) ;
#9801=CIRCLE ( 'NONE', #2992, 1.499999999999994449 ) ;
#9806=AXIS2_PLACEMENT_3D ( 'NONE', #12571, #2889, #486 ) ;
#9812=VERTEX_POINT ( 'NONE', #9492 ) ;
#9814=VECTOR ( 'NONE', #12287, 1000.000000000000000 ) ;
#9815=CIRCLE ( 'NONE', #9529, 1.000000000000000888 ) ;
#9817=ORIENTED_EDGE ( 'NONE', *, *, #12839, .T. ) ;
#9833=EDGE_CURVE ( 'NONE', #1592, #11107, #3640, .T. ) ;
#9836=AXIS2_PLACEMENT_3D ( 'NONE', #5735, #8124, #5811 ) ;
#9841=TOROIDAL_SURFACE ( 'NONE', #14851, 1.000000000000000000, 0.5000000000000000000 ) ;
#9842=EDGE_CURVE ( 'NONE', #5777, #7205, #10753, .T. ) ;
#9845=DIRECTION ( 'NONE',  ( 0.000000000000000000, -0.9902680687415712502, -0.1391731009600586100 ) ) ;
#9850=ORIENTED_EDGE ( 'NONE', *, *, #6019, .F. ) ;
#9853=EDGE_CURVE ( 'NONE', #10500, #10070, #10600, .T. ) ;
#9858=CARTESIAN_POINT ( 'NONE',  ( -63.50000000000002842, 15.17911304468680100, 9.062306170389884841 ) ) ;
#9861=DIRECTION ( 'NONE',  ( -0.000000000000000000, -0.9902680687415712502, -0.1391731009600586100 ) ) ;
#9862=VECTOR ( 'NONE', #9495, 1000.000000000000000 ) ;
#9866=AXIS2_PLACEMENT_3D ( 'NONE', #2135, #5698, #14131 ) ;
#9867=ORIENTED_EDGE ( 'NONE', *, *, #5187, .F. ) ;
#9869=LINE ( 'NONE', #12218, #3085 ) ;
#9873=CARTESIAN_POINT ( 'NONE',  ( 184.0000000000000568, -201.3058001507315566, 76.45141194869098911 ) ) ;
#9874=DIRECTION ( 'NONE',  ( -0.000000000000000000, -0.000000000000000000, -1.000000000000000000 ) ) ;
#9876=VECTOR ( 'NONE', #11742, 1000.000000000000000 ) ;
#9877=LINE ( 'NONE', #14896, #10434 ) ;
#9879=CARTESIAN_POINT ( 'NONE',  ( 190.0000000000000853, -179.3058001507315566, 64.88378295107887084 ) ) ;
#9881=ORIENTED_EDGE ( 'NONE', *, *, #11392, .T. ) ;
#9886=AXIS2_PLACEMENT_3D ( 'NONE', #3153, #7987, #12773 ) ;
#9887=ORIENTED_EDGE ( 'NONE', *, *, #13066, .T. ) ;
#9889=DIRECTION ( 'NONE',  ( -0.000000000000000000, 1.000000000000000000, 6.938893903907227145E-17 ) ) ;
#9891=EDGE_CURVE ( 'NONE', #11360, #3344, #1033, .T. ) ;
#9894=AXIS2_PLACEMENT_3D ( 'NONE', #11128, #7424, #2516 ) ;
#9900=FACE_OUTER_BOUND ( 'NONE', #10325, .T. ) ;
#9901=ORIENTED_EDGE ( 'NONE', *, *, #12268, .T. ) ;
#9902=ORIENTED_EDGE ( 'NONE', *, *, #2443, .T. ) ;
#9907=FACE_OUTER_BOUND ( 'NONE', #1772, .T. ) ;
#9908=DIRECTION ( 'NONE',  ( 1.000000000000000000, -2.751328491981765035E-32, 3.965082230804130220E-16 ) ) ;
#9911=FACE_OUTER_BOUND ( 'NONE', #729, .T. ) ;
#9919=DIRECTION ( 'NONE',  ( 0.000000000000000000, 0.1391731009600592484, -0.9902680687415712502 ) ) ;
#9922=AXIS2_PLACEMENT_3D ( 'NONE', #5613, #7993, #1964 ) ;
#9926=EDGE_LOOP ( 'NONE', ( #13499, #8988, #15486, #2983 ) ) ;
#9929=CARTESIAN_POINT ( 'NONE',  ( -64.00000000000002842, -179.3058001507315851, 64.88378295107887084 ) ) ;
#9934=ADVANCED_FACE ( 'NONE', ( #12083 ), #10516, .F. ) ;
#9937=DIRECTION ( 'NONE',  ( 0.000000000000000000, 0.000000000000000000, -1.000000000000000000 ) ) ;
#9938=CARTESIAN_POINT ( 'NONE',  ( 190.5000000000000568, 16.03993994372673981, -3.075184203610571654 ) ) ;
#9939=EDGE_LOOP ( 'NONE', ( #7571, #3481, #2091, #5132 ) ) ;
#9942=ORIENTED_EDGE ( 'NONE', *, *, #5440, .T. ) ;
#9951=ORIENTED_EDGE ( 'NONE', *, *, #2540, .F. ) ;
#9952=EDGE_CURVE ( 'NONE', #101, #227, #947, .T. ) ;
#9957=CIRCLE ( 'NONE', #4642, 0.9999999999999991118 ) ;
#9959=CARTESIAN_POINT ( 'NONE',  ( -76.00000000000001421, 15.10952649420676863, 9.557440204760682789 ) ) ;
#9964=FACE_OUTER_BOUND ( 'NONE', #4504, .T. ) ;
#9965=ORIENTED_EDGE ( 'NONE', *, *, #6762, .F. ) ;
#9970=CARTESIAN_POINT ( 'NONE',  ( -64.00000000000002842, -178.6666270497714777, 53.18093594598651919 ) ) ;
#9972=ADVANCED_FACE ( 'NONE', ( #9964 ), #1547, .T. ) ;
#9975=DIRECTION ( 'NONE',  ( -1.000000000000000000, -6.938893903907222067E-15, 0.000000000000000000 ) ) ;
#9978=CARTESIAN_POINT ( 'NONE',  ( -70.00000000000000000, 17.53993994372673981, -10.99999999999999645 ) ) ;
#9979=CIRCLE ( 'NONE', #3661, 0.5000000000000004441 ) ;
#9981=ORIENTED_EDGE ( 'NONE', *, *, #2082, .T. ) ;
#9993=DIRECTION ( 'NONE',  ( 0.000000000000000000, 0.1391731009600592484, -0.9902680687415712502 ) ) ;
#9996=LINE ( 'NONE', #13761, #2304 ) ;
#9999=CARTESIAN_POINT ( 'NONE',  ( 178.0000000000000853, 15.03993994372673804, 38.07518420361041933 ) ) ;
#10004=ORIENTED_EDGE ( 'NONE', *, *, #3664, .T. ) ;
#10017=ORIENTED_EDGE ( 'NONE', *, *, #15336, .T. ) ;
#10021=LINE ( 'NONE', #13873, #9814 ) ;
#10022=CARTESIAN_POINT ( 'NONE',  ( 190.5000000000000568, -178.8753867012115961, 64.82329228561619061 ) ) ;
#10028=DIRECTION ( 'NONE',  ( -0.000000000000000000, 1.000000000000000000, -0.000000000000000000 ) ) ;
#10029=DIRECTION ( 'NONE',  ( -0.000000000000000000, 0.000000000000000000, -1.000000000000000000 ) ) ;
#10031=ORIENTED_EDGE ( 'NONE', *, *, #1542, .F. ) ;
#10036=VERTEX_POINT ( 'NONE', #4247 ) ;
#10040=CARTESIAN_POINT ( 'NONE',  ( 190.5000000000000568, 15.53993994372673981, 10.05257423913146475 ) ) ;
#10041=ORIENTED_EDGE ( 'NONE', *, *, #3994, .T. ) ;
#10042=CIRCLE ( 'NONE', #9033, 0.5000000000000004441 ) ;
#10049=LINE ( 'NONE', #313, #8320 ) ;
#10051=ORIENTED_EDGE ( 'NONE', *, *, #1897, .F. ) ;
#10052=CARTESIAN_POINT ( 'NONE',  ( -64.00000000000002842, 15.53993994372673626, 52.49999999999997868 ) ) ;
#10054=CIRCLE ( 'NONE', #15565, 0.5000000000000004441 ) ;
#10055=ORIENTED_EDGE ( 'NONE', *, *, #6451, .F. ) ;
#10058=EDGE_CURVE ( 'NONE', #7982, #9410, #9241, .T. ) ;
#10059=CYLINDRICAL_SURFACE ( 'NONE', #6038, 0.5000000000000004441 ) ;
#10063=CIRCLE ( 'NONE', #3250, 0.5000000000000004441 ) ;
#10069=LINE ( 'NONE', #6525, #5012 ) ;
#10070=VERTEX_POINT ( 'NONE', #532 ) ;
#10074=AXIS2_PLACEMENT_3D ( 'NONE', #3898, #1679, #7537 ) ;
#10075=CIRCLE ( 'NONE', #13837, 1.000000000000000000 ) ;
#10080=AXIS2_PLACEMENT_3D ( 'NONE', #4235, #14809, #9073 ) ;
#10083=CIRCLE ( 'NONE', #740, 1.499999999999997780 ) ;
#10086=CARTESIAN_POINT ( 'NONE',  ( 177.5000000000000853, 14.90076684276667862, 37.08491613486885541 ) ) ;
#10095=CARTESIAN_POINT ( 'NONE',  ( 178.0000000000000853, 15.53993994372673804, 38.07518420361041933 ) ) ;
#10098=DIRECTION ( 'NONE',  ( 1.000000000000000000, -0.000000000000000000, -0.000000000000000000 ) ) ;
#10101=EDGE_CURVE ( 'NONE', #12639, #7344, #4318, .T. ) ;
#10102=ORIENTED_EDGE ( 'NONE', *, *, #4971, .F. ) ;
#10103=AXIS2_PLACEMENT_3D ( 'NONE', #4986, #145, #14524 ) ;
#10116=ADVANCED_FACE ( 'NONE', ( #686 ), #15152, .T. ) ;
#10117=PLANE ( 'NONE',  #4383 ) ;
#10118=CARTESIAN_POINT ( 'NONE',  ( 190.5000000000000568, 15.03993994372673981, -3.075184203610571654 ) ) ;
#10120=AXIS2_PLACEMENT_3D ( 'NONE', #10790, #8508, #9452 ) ;
#10121=DIRECTION ( 'NONE',  ( 0.000000000000000000, 0.000000000000000000, -1.000000000000000000 ) ) ;
#10124=VERTEX_POINT ( 'NONE', #7912 ) ;
#10126=ORIENTED_EDGE ( 'NONE', *, *, #10920, .T. ) ;
#10127=CARTESIAN_POINT ( 'NONE',  ( -70.00000000000000000, 17.53993994372673981, -12.49999999999999289 ) ) ;
#10130=CARTESIAN_POINT ( 'NONE',  ( 190.0000000000000568, -179.3058001507315566, -17.76585208085566947 ) ) ;
#10133=CIRCLE ( 'NONE', #11886, 0.5000000000000004441 ) ;
#10136=ORIENTED_EDGE ( 'NONE', *, *, #4399, .T. ) ;
#10139=CARTESIAN_POINT ( 'NONE',  ( -63.50000000000002842, 15.47035339324670922, 37.00486596562913633 ) ) ;
#10140=CARTESIAN_POINT ( 'NONE',  ( 178.0000000000000853, -178.8058001507315566, -17.19066787724516843 ) ) ;
#10142=VECTOR ( 'NONE', #12460, 1000.000000000000000 ) ;
#10143=CARTESIAN_POINT ( 'NONE',  ( 190.5000000000000853, -179.8058001507315566, 52.76585208085545275 ) ) ;
#10150=ORIENTED_EDGE ( 'NONE', *, *, #10794, .T. ) ;
#10155=LINE ( 'NONE', #9929, #13455 ) ;
#10156=CARTESIAN_POINT ( 'NONE',  ( 177.5000000000000853, -179.3058001507315566, -17.19066787724516843 ) ) ;
#10158=ADVANCED_FACE ( 'NONE', ( #9170 ), #13969, .T. ) ;
#10164=CARTESIAN_POINT ( 'NONE',  ( 190.0000000000000853, -178.8753867012115961, 64.82329228561619061 ) ) ;
#10168=TOROIDAL_SURFACE ( 'NONE', #14935, 1.000000000000000000, 0.5000000000000000000 ) ;
#10172=CYLINDRICAL_SURFACE ( 'NONE', #10822, 0.5000000000000004441 ) ;
#10175=FACE_BOUND ( 'NONE', #8091, .T. ) ;
#10181=EDGE_CURVE ( 'NONE', #6887, #14401, #3072, .T. ) ;
#10186=CIRCLE ( 'NONE', #6674, 0.5000000000000004441 ) ;
#10191=CIRCLE ( 'NONE', #9436, 0.5000000000000004441 ) ;
#10193=APPLICATION_CONTEXT ( 'automotive_design' ) ;
#10194=CARTESIAN_POINT ( 'NONE',  ( -64.00000000000002842, -178.8058001507315566, 52.19066787724494816 ) ) ;
#10201=VERTEX_POINT ( 'NONE', #6955 ) ;
#10207=FACE_BOUND ( 'NONE', #14659, .T. ) ;
#10209=ORIENTED_EDGE ( 'NONE', *, *, #11823, .T. ) ;
#10212=CARTESIAN_POINT ( 'NONE',  ( 184.0000000000000568, 17.53993994372673626, 47.49999999999997868 ) ) ;
#10218=CARTESIAN_POINT ( 'NONE',  ( 177.5000000000000853, -179.3058001507315566, 65.31842631998698323 ) ) ;
#10220=VECTOR ( 'NONE', #4364, 1000.000000000000000 ) ;
#10221=CARTESIAN_POINT ( 'NONE',  ( 178.0000000000000853, 16.03993994372673981, 7.553451883674125344E-16 ) ) ;
#10222=EDGE_LOOP ( 'NONE', ( #9605, #9011, #10389, #1170 ) ) ;
#10233=CIRCLE ( 'NONE', #6467, 1.000000000000000888 ) ;
#10235=EDGE_CURVE ( 'NONE', #13797, #9039, #11762, .T. ) ;
#10236=CYLINDRICAL_SURFACE ( 'NONE', #8627, 0.5000000000000001110 ) ;
#10237=ORIENTED_EDGE ( 'NONE', *, *, #9332, .F. ) ;
#10238=DIRECTION ( 'NONE',  ( 1.000000000000000000, 0.000000000000000000, 0.000000000000000000 ) ) ;
#10248=PLANE ( 'NONE',  #177 ) ;
#10253=AXIS2_PLACEMENT_3D ( 'NONE', #3862, #285, #6396 ) ;
#10254=AXIS2_PLACEMENT_3D ( 'NONE', #9460, #8365, #11825 ) ;
#10261=ORIENTED_EDGE ( 'NONE', *, *, #4084, .T. ) ;
#10267=FACE_BOUND ( 'NONE', #12503, .T. ) ;
#10270=CARTESIAN_POINT ( 'NONE',  ( 178.0000000000000853, 16.03993994372673981, 24.94742576086838781 ) ) ;
#10275=DIRECTION ( 'NONE',  ( 0.000000000000000000, 0.1391731009600592484, 0.9902680687415712502 ) ) ;
#10276=EDGE_LOOP ( 'NONE', ( #14517, #8750, #8315, #1922 ) ) ;
#10277=DIRECTION ( 'NONE',  ( 0.000000000000000000, 0.000000000000000000, -1.000000000000000000 ) ) ;
#10280=ORIENTED_EDGE ( 'NONE', *, *, #14988, .T. ) ;
#10284=ORIENTED_EDGE ( 'NONE', *, *, #3586, .F. ) ;
#10298=VERTEX_POINT ( 'NONE', #9318 ) ;
#10310=DIRECTION ( 'NONE',  ( -1.000000000000000000, 0.000000000000000000, 0.000000000000000000 ) ) ;
#10311=EDGE_CURVE ( 'NONE', #15212, #4169, #2202, .T. ) ;
#10320=CARTESIAN_POINT ( 'NONE',  ( -64.00000000000002842, -178.8058001507315566, -30.31842631998718574 ) ) ;
#10321=EDGE_LOOP ( 'NONE', ( #5587, #12171, #12712, #12251 ) ) ;
#10324=EDGE_CURVE ( 'NONE', #14668, #4290, #3317, .T. ) ;
#10325=EDGE_LOOP ( 'NONE', ( #12262, #7743, #1935, #9350 ) ) ;
#10326=ORIENTED_EDGE ( 'NONE', *, *, #4176, .T. ) ;
#10328=CARTESIAN_POINT ( 'NONE',  ( 184.0000000000000568, -181.3058001507315566, 76.45141194869098911 ) ) ;
#10336=FACE_OUTER_BOUND ( 'NONE', #14285, .T. ) ;
#10339=DIRECTION ( 'NONE',  ( -0.000000000000000000, 6.938893903907227145E-17, -1.000000000000000000 ) ) ;
#10340=VERTEX_POINT ( 'NONE', #7268 ) ;
#10344=CIRCLE ( 'NONE', #3535, 0.5000000000000004441 ) ;
#10346=FACE_OUTER_BOUND ( 'NONE', #1846, .T. ) ;
#10349=CARTESIAN_POINT ( 'NONE',  ( -76.00000000000001421, -179.3058001507315566, -17.19066787724516843 ) ) ;
#10356=CARTESIAN_POINT ( 'NONE',  ( 178.0000000000000853, -178.8058001507315566, -17.19066787724516843 ) ) ;
#10361=DIRECTION ( 'NONE',  ( 0.000000000000000000, -0.1391731009600660485, -0.9902680687415702510 ) ) ;
#10364=ORIENTED_EDGE ( 'NONE', *, *, #7671, .T. ) ;
#10366=DIRECTION ( 'NONE',  ( 0.000000000000000000, 0.000000000000000000, -1.000000000000000000 ) ) ;
#10367=DIRECTION ( 'NONE',  ( 1.000000000000000000, 0.000000000000000000, 0.000000000000000000 ) ) ;
#10371=CIRCLE ( 'NONE', #1034, 0.5000000000000069944 ) ;
#10375=DIRECTION ( 'NONE',  ( 0.000000000000000000, 0.000000000000000000, 1.000000000000000000 ) ) ;
#10376=EDGE_CURVE ( 'NONE', #2480, #10747, #6156, .T. ) ;
#10386=AXIS2_PLACEMENT_3D ( 'NONE', #9625, #5989, #1160 ) ;
#10387=FACE_BOUND ( 'NONE', #14172, .T. ) ;
#10389=ORIENTED_EDGE ( 'NONE', *, *, #7218, .F. ) ;
#10390=AXIS2_PLACEMENT_3D ( 'NONE', #8693, #13483, #1568 ) ;
#10391=CYLINDRICAL_SURFACE ( 'NONE', #2899, 0.5000000000000001110 ) ;
#10393=EDGE_CURVE ( 'NONE', #13605, #8345, #11042, .T. ) ;
#10394=EDGE_CURVE ( 'NONE', #12187, #4995, #6878, .T. ) ;
#10396=DIRECTION ( 'NONE',  ( 0.000000000000000000, 1.000000000000000000, 0.000000000000000000 ) ) ;
#10397=VECTOR ( 'NONE', #8597, 1000.000000000000000 ) ;
#10398=LINE ( 'NONE', #11578, #12838 ) ;
#10402=ORIENTED_EDGE ( 'NONE', *, *, #1077, .T. ) ;
#10408=DIRECTION ( 'NONE',  ( 0.000000000000000000, 0.000000000000000000, -1.000000000000000000 ) ) ;
#10414=DIRECTION ( 'NONE',  ( 0.000000000000000000, 0.000000000000000000, -1.000000000000000000 ) ) ;
#10418=EDGE_LOOP ( 'NONE', ( #2709, #6604, #9256, #15016 ) ) ;
#10419=DIRECTION ( 'NONE',  ( 0.000000000000000000, -1.000000000000000000, -4.956352788505162775E-17 ) ) ;
#10421=AXIS2_PLACEMENT_3D ( 'NONE', #6945, #9161, #6641 ) ;
#10426=AXIS2_PLACEMENT_3D ( 'NONE', #8283, #13062, #15200 ) ;
#10428=EDGE_CURVE ( 'NONE', #3793, #13203, #9869, .T. ) ;
#10429=DIRECTION ( 'NONE',  ( 0.000000000000000000, 1.000000000000000000, 6.938893903907227145E-17 ) ) ;
#10433=ORIENTED_EDGE ( 'NONE', *, *, #6575, .F. ) ;
#10434=VECTOR ( 'NONE', #1483, 1000.000000000000000 ) ;
#10439=AXIS2_PLACEMENT_3D ( 'NONE', #11494, #5798, #10534 ) ;
#10449=DIRECTION ( 'NONE',  ( -1.000000000000000000, -0.000000000000000000, -0.000000000000000000 ) ) ;
#10450=EDGE_CURVE ( 'NONE', #13870, #7084, #194, .T. ) ;
#10452=CIRCLE ( 'NONE', #10962, 0.5000000000000004441 ) ;
#10463=VERTEX_POINT ( 'NONE', #1241 ) ;
#10464=EDGE_CURVE ( 'NONE', #5369, #3026, #3326, .T. ) ;
#10468=AXIS2_PLACEMENT_3D ( 'NONE', #4382, #7801, #10238 ) ;
#10472=CARTESIAN_POINT ( 'NONE',  ( 190.0000000000000568, -179.8058001507315566, -30.31842631998718574 ) ) ;
#10474=DIRECTION ( 'NONE',  ( 0.000000000000000000, -1.000000000000000000, -6.938893903907227145E-17 ) ) ;
#10476=LINE ( 'NONE', #10630, #8535 ) ;
#10478=ORIENTED_EDGE ( 'NONE', *, *, #1989, .F. ) ;
#10480=ORIENTED_EDGE ( 'NONE', *, *, #4971, .T. ) ;
#10482=DIRECTION ( 'NONE',  ( 0.000000000000000000, -1.000000000000000000, -6.938893903907222067E-15 ) ) ;
#10492=EDGE_CURVE ( 'NONE', #11360, #6077, #5098, .T. ) ;
#10494=VECTOR ( 'NONE', #5006, 1000.000000000000000 ) ;
#10496=CARTESIAN_POINT ( 'NONE',  ( 178.0000000000000853, 11.87216911405866959, 26.40245448993442068 ) ) ;
#10498=ORIENTED_EDGE ( 'NONE', *, *, #5403, .T. ) ;
#10500=VERTEX_POINT ( 'NONE', #2762 ) ;
#10501=FACE_OUTER_BOUND ( 'NONE', #1830, .T. ) ;
#10502=CARTESIAN_POINT ( 'NONE',  ( 177.5000000000000853, 16.03993994372673981, -3.075184203610571654 ) ) ;
#10503=AXIS2_PLACEMENT_3D ( 'NONE', #2423, #7179, #5979 ) ;
#10504=EDGE_CURVE ( 'NONE', #11537, #10667, #9003, .T. ) ;
#10507=ORIENTED_EDGE ( 'NONE', *, *, #2003, .T. ) ;
#10513=ORIENTED_EDGE ( 'NONE', *, *, #8761, .T. ) ;
#10514=ORIENTED_EDGE ( 'NONE', *, *, #3537, .F. ) ;
#10516=CYLINDRICAL_SURFACE ( 'NONE', #13138, 0.5000000000000004441 ) ;
#10517=EDGE_CURVE ( 'NONE', #14746, #2220, #5609, .T. ) ;
#10518=EDGE_LOOP ( 'NONE', ( #13098, #12244, #10051, #6187 ) ) ;
#10524=DIRECTION ( 'NONE',  ( -0.000000000000000000, 0.9902680687415712502, 0.1391731009600584990 ) ) ;
#10525=CARTESIAN_POINT ( 'NONE',  ( 190.0000000000000568, -178.8058001507315566, -17.19066787724516843 ) ) ;
#10526=CARTESIAN_POINT ( 'NONE',  ( -70.00000000000000000, 15.53993994372673981, -12.49999999999999289 ) ) ;
#10532=ORIENTED_EDGE ( 'NONE', *, *, #7803, .T. ) ;
#10533=EDGE_CURVE ( 'NONE', #4972, #2866, #3838, .T. ) ;
#10534=DIRECTION ( 'NONE',  ( 0.000000000000000000, 0.000000000000000000, -1.000000000000000000 ) ) ;
#10536=CARTESIAN_POINT ( 'NONE',  ( 190.0000000000000853, 15.03993994372673804, 38.07518420361041933 ) ) ;
#10537=AXIS2_PLACEMENT_3D ( 'NONE', #10328, #4155, #1791 ) ;
#10541=CARTESIAN_POINT ( 'NONE',  ( -64.00000000000002842, -179.3058001507315566, -29.88378295107905913 ) ) ;
#10543=ORIENTED_EDGE ( 'NONE', *, *, #12780, .F. ) ;
#10546=LINE ( 'NONE', #8275, #707 ) ;
#10550=EDGE_CURVE ( 'NONE', #6887, #9678, #2071, .T. ) ;
#10552=VERTEX_POINT ( 'NONE', #14816 ) ;
#10564=ADVANCED_FACE ( 'NONE', ( #6485 ), #533, .T. ) ;
#10567=VECTOR ( 'NONE', #12498, 1000.000000000000114 ) ;
#10568=CARTESIAN_POINT ( 'NONE',  ( -63.50000000000002842, -181.3058001507315566, 84.88378295107885663 ) ) ;
#10569=CARTESIAN_POINT ( 'NONE',  ( 184.0000000000000568, -179.3058001507315566, -42.95141194869119516 ) ) ;
#10576=CARTESIAN_POINT ( 'NONE',  ( -64.00000000000002842, -179.8058001507315566, -30.31842631998718574 ) ) ;
#10577=CARTESIAN_POINT ( 'NONE',  ( 177.5000000000000853, -178.8058001507315566, -30.31842631998718574 ) ) ;
#10579=VECTOR ( 'NONE', #14078, 1000.000000000000000 ) ;
#10581=CARTESIAN_POINT ( 'NONE',  ( 184.0000000000000568, 15.53993994372673626, 45.99999999999998579 ) ) ;
#10583=CIRCLE ( 'NONE', #12577, 0.5000000000000004441 ) ;
#10585=AXIS2_PLACEMENT_3D ( 'NONE', #10221, #6600, #801 ) ;
#10590=DIRECTION ( 'NONE',  ( 1.000000000000000000, 0.000000000000000000, 0.000000000000000000 ) ) ;
#10592=EDGE_CURVE ( 'NONE', #1358, #7962, #5653, .T. ) ;
#10594=FACE_OUTER_BOUND ( 'NONE', #11718, .T. ) ;
#10596=DIRECTION ( 'NONE',  ( 0.000000000000000000, -0.1391731009600660485, -0.9902680687415702510 ) ) ;
#10597=EDGE_LOOP ( 'NONE', ( #4690, #1789, #9358, #682 ) ) ;
#10599=DIRECTION ( 'NONE',  ( 1.000000000000000000, -2.751328491981765035E-32, 3.965082230804130220E-16 ) ) ;
#10600=LINE ( 'NONE', #7292, #14883 ) ;
#10602=DIRECTION ( 'NONE',  ( 0.000000000000000000, 0.9902680687415712502, 0.1391731009600596092 ) ) ;
#10603=AXIS2_PLACEMENT_3D ( 'NONE', #14556, #9190, #12955 ) ;
#10604=AXIS2_PLACEMENT_3D ( 'NONE', #15429, #4627, #7968 ) ;
#10605=CARTESIAN_POINT ( 'NONE',  ( -70.00000000000000000, -179.3058001507315566, -42.95141194869119516 ) ) ;
#10606=EDGE_LOOP ( 'NONE', ( #8601, #6906, #14438, #2297 ) ) ;
#10607=EDGE_CURVE ( 'NONE', #7205, #3793, #12400, .T. ) ;
#10614=CARTESIAN_POINT ( 'NONE',  ( 175.9483885134608272, -178.8058001507315566, 52.19066787724494816 ) ) ;
#10619=DIRECTION ( 'NONE',  ( -1.000000000000000000, 0.000000000000000000, 0.000000000000000000 ) ) ;
#10622=TOROIDAL_SURFACE ( 'NONE', #13624, 1.000000000000000000, 0.5000000000000000000 ) ;
#10624=EDGE_LOOP ( 'NONE', ( #10824, #9489, #15196, #12 ) ) ;
#10630=CARTESIAN_POINT ( 'NONE',  ( 190.0000000000000853, 15.53993994372673804, 52.49999999999997868 ) ) ;
#10634=ORIENTED_EDGE ( 'NONE', *, *, #2581, .T. ) ;
#10636=DIRECTION ( 'NONE',  ( 0.000000000000000000, 0.000000000000000000, 1.000000000000000000 ) ) ;
#10637=CARTESIAN_POINT ( 'NONE',  ( 190.5000000000000568, 16.03993994372673981, 9.617930870223348805 ) ) ;
#10650=CARTESIAN_POINT ( 'NONE',  ( 178.0000000000000853, 15.03993994372673804, 37.07518420361041933 ) ) ;
#10655=ORIENTED_EDGE ( 'NONE', *, *, #12780, .T. ) ;
#10664=EDGE_CURVE ( 'NONE', #5844, #13203, #1562, .T. ) ;
#10667=VERTEX_POINT ( 'NONE', #7799 ) ;
#10671=DIRECTION ( 'NONE',  ( -0.000000000000000000, 0.000000000000000000, 1.000000000000000000 ) ) ;
#10674=DIRECTION ( 'NONE',  ( 1.000000000000000000, -2.751328491981765035E-32, 3.965082230804130220E-16 ) ) ;
#10676=AXIS2_PLACEMENT_3D ( 'NONE', #14579, #8605, #3780 ) ;
#10678=FACE_OUTER_BOUND ( 'NONE', #13679, .T. ) ;
#10682=EDGE_CURVE ( 'NONE', #6077, #13452, #14664, .T. ) ;
#10683=ADVANCED_FACE ( 'NONE', ( #13858 ), #10236, .T. ) ;
#10689=DIRECTION ( 'NONE',  ( 1.000000000000000000, 0.000000000000000000, 0.000000000000000000 ) ) ;
#10690=DIRECTION ( 'NONE',  ( -1.000000000000000000, -0.000000000000000000, -0.000000000000000000 ) ) ;
#10691=CARTESIAN_POINT ( 'NONE',  ( 178.0000000000000853, -179.3058001507315851, 64.88378295107887084 ) ) ;
#10692=ORIENTED_EDGE ( 'NONE', *, *, #15288, .F. ) ;
#10698=DIRECTION ( 'NONE',  ( 0.000000000000000000, 0.000000000000000000, 1.000000000000000000 ) ) ;
#10702=VECTOR ( 'NONE', #3686, 1000.000000000000114 ) ;
#10705=ORIENTED_EDGE ( 'NONE', *, *, #11020, .T. ) ;
#10706=CARTESIAN_POINT ( 'NONE',  ( -61.94838851346079167, -181.3058001507315566, 84.88378295107885663 ) ) ;
#10708=DIRECTION ( 'NONE',  ( 0.000000000000000000, -0.9902680687415711391, 0.1391731009600603308 ) ) ;
#10713=CARTESIAN_POINT ( 'NONE',  ( 177.5000000000000853, 16.03993994372673626, 52.49999999999997868 ) ) ;
#10715=ADVANCED_FACE ( 'NONE', ( #1135 ), #7634, .T. ) ;
#10717=CYLINDRICAL_SURFACE ( 'NONE', #336, 0.5000000000000004441 ) ;
#10723=DIRECTION ( 'NONE',  ( 0.000000000000000000, -1.000000000000000000, -4.956352788505160310E-17 ) ) ;
#10724=VECTOR ( 'NONE', #10689, 1000.000000000000000 ) ;
#10732=DIRECTION ( 'NONE',  ( -0.000000000000000000, 1.000000000000000000, -0.000000000000000000 ) ) ;
#10733=CARTESIAN_POINT ( 'NONE',  ( -64.00000000000002842, -179.3058001507315566, 84.88378295107887084 ) ) ;
#10744=ORIENTED_EDGE ( 'NONE', *, *, #5991, .T. ) ;
#10747=VERTEX_POINT ( 'NONE', #3592 ) ;
#10748=CYLINDRICAL_SURFACE ( 'NONE', #6462, 0.5000000000000000000 ) ;
#10751=VERTEX_POINT ( 'NONE', #8199 ) ;
#10753=LINE ( 'NONE', #4827, #2300 ) ;
#10758=CARTESIAN_POINT ( 'NONE',  ( -70.00000000000000000, 15.53993994372673626, 47.49999999999997868 ) ) ;
#10763=VERTEX_POINT ( 'NONE', #11733 ) ;
#10764=EDGE_CURVE ( 'NONE', #12538, #3389, #5728, .T. ) ;
#10767=DIRECTION ( 'NONE',  ( -0.000000000000000000, -6.938893903907227145E-17, 1.000000000000000000 ) ) ;
#10768=ORIENTED_EDGE ( 'NONE', *, *, #15388, .T. ) ;
#10772=VERTEX_POINT ( 'NONE', #9367 ) ;
#10775=CIRCLE ( 'NONE', #5730, 0.5000000000000069944 ) ;
#10780=ORIENTED_EDGE ( 'NONE', *, *, #4444, .T. ) ;
#10783=ORIENTED_EDGE ( 'NONE', *, *, #921, .T. ) ;
#10784=LINE ( 'NONE', #13447, #6352 ) ;
#10787=CARTESIAN_POINT ( 'NONE',  ( 190.5000000000000853, 15.17911304468679745, 25.93769382960994818 ) ) ;
#10790=CARTESIAN_POINT ( 'NONE',  ( -64.00000000000002842, 23.05038067821381986, -0.9395626039331514967 ) ) ;
#10794=EDGE_CURVE ( 'NONE', #4995, #2689, #6636, .T. ) ;
#10807=AXIS2_PLACEMENT_3D ( 'NONE', #8954, #3893, #12556 ) ;
#10812=AXIS2_PLACEMENT_3D ( 'NONE', #1893, #6950, #11757 ) ;
#10819=MANIFOLD_SOLID_BREP ( 'Mirror1', #3342 ) ;
#10822=AXIS2_PLACEMENT_3D ( 'NONE', #5118, #1790, #6630 ) ;
#10824=ORIENTED_EDGE ( 'NONE', *, *, #8290, .F. ) ;
#10826=ADVANCED_FACE ( 'NONE', ( #14702 ), #6203, .T. ) ;
#10827=ORIENTED_EDGE ( 'NONE', *, *, #8331, .T. ) ;
#10831=ORIENTED_EDGE ( 'NONE', *, *, #9435, .F. ) ;
#10847=CARTESIAN_POINT ( 'NONE',  ( -63.50000000000002842, 15.03993994372673804, 38.07518420361041933 ) ) ;
#10848=EDGE_CURVE ( 'NONE', #9239, #6280, #165, .T. ) ;
#10849=LINE ( 'NONE', #4, #5697 ) ;
#10853=VERTEX_POINT ( 'NONE', #3830 ) ;
#10862=AXIS2_PLACEMENT_3D ( 'NONE', #2144, #3177, #10366 ) ;
#10863=ORIENTED_EDGE ( 'NONE', *, *, #2088, .T. ) ;
#10864=AXIS2_PLACEMENT_3D ( 'NONE', #15194, #1936, #4388 ) ;
#10872=DIRECTION ( 'NONE',  ( 0.000000000000000000, 0.000000000000000000, -1.000000000000000000 ) ) ;
#10875=CYLINDRICAL_SURFACE ( 'NONE', #10120, 0.5000000000000001110 ) ;
#10882=CARTESIAN_POINT ( 'NONE',  ( -76.00000000000001421, 15.17911304468679923, 9.062306170389897275 ) ) ;
#10890=VECTOR ( 'NONE', #10732, 1000.000000000000000 ) ;
#10891=DIRECTION ( 'NONE',  ( -1.000000000000000000, 0.000000000000000000, 0.000000000000000000 ) ) ;
#10894=CARTESIAN_POINT ( 'NONE',  ( -70.00000000000000000, 15.53993994372673981, -13.99999999999999112 ) ) ;
#10895=VERTEX_POINT ( 'NONE', #13921 ) ;
#10903=DIRECTION ( 'NONE',  ( -1.000000000000000000, 0.000000000000000000, 0.000000000000000000 ) ) ;
#10909=CARTESIAN_POINT ( 'NONE',  ( -63.50000000000002842, -178.8058001507315566, -17.19066787724516843 ) ) ;
#10914=LINE ( 'NONE', #14366, #3008 ) ;
#10918=CARTESIAN_POINT ( 'NONE',  ( -61.94838851346079167, 15.03993994372673981, -3.075184203610571654 ) ) ;
#10919=DIRECTION ( 'NONE',  ( 0.000000000000000000, 1.000000000000000000, 6.938893903907227145E-17 ) ) ;
#10920=EDGE_CURVE ( 'NONE', #4028, #12308, #719, .T. ) ;
#10923=AXIS2_PLACEMENT_3D ( 'NONE', #8775, #12396, #10121 ) ;
#10924=ORIENTED_EDGE ( 'NONE', *, *, #5935, .F. ) ;
#10926=ORIENTED_EDGE ( 'NONE', *, *, #13091, .F. ) ;
#10927=CIRCLE ( 'NONE', #14967, 0.5000000000000004441 ) ;
#10930=ORIENTED_EDGE ( 'NONE', *, *, #12087, .T. ) ;
#10931=EDGE_LOOP ( 'NONE', ( #4625, #13011, #1728, #11008, #5813 ) ) ;
#10934=ORIENTED_EDGE ( 'NONE', *, *, #1926, .T. ) ;
#10935=EDGE_CURVE ( 'NONE', #10667, #4671, #14606, .T. ) ;
#10941=ADVANCED_FACE ( 'NONE', ( #6827 ), #9197, .T. ) ;
#10945=CARTESIAN_POINT ( 'NONE',  ( -64.00000000000002842, -178.8058001507315566, 65.31842631998698323 ) ) ;
#10946=DIRECTION ( 'NONE',  ( 0.000000000000000000, 0.1391731009600660485, -0.9902680687415702510 ) ) ;
#10949=ADVANCED_FACE ( 'NONE', ( #15089 ), #9327, .T. ) ;
#10960=DIRECTION ( 'NONE',  ( 0.000000000000000000, -1.000000000000000000, 0.000000000000000000 ) ) ;
#10961=CARTESIAN_POINT ( 'NONE',  ( 184.0000000000000568, 15.53993994372673981, -13.99999999999999112 ) ) ;
#10962=AXIS2_PLACEMENT_3D ( 'NONE', #4724, #14662, #1474 ) ;
#10966=CARTESIAN_POINT ( 'NONE',  ( 178.0000000000000853, -179.3058001507315566, -17.76585208085566947 ) ) ;
#10968=ORIENTED_EDGE ( 'NONE', *, *, #11334, .F. ) ;
#10971=VERTEX_POINT ( 'NONE', #1914 ) ;
#10973=CARTESIAN_POINT ( 'NONE',  ( -76.00000000000001421, -179.3058001507315566, -51.45141194869120937 ) ) ;
#10987=ORIENTED_EDGE ( 'NONE', *, *, #6979, .F. ) ;
#10994=CARTESIAN_POINT ( 'NONE',  ( 177.5000000000000853, -178.9449732516916072, 64.32815825124541220 ) ) ;
#11001=CARTESIAN_POINT ( 'NONE',  ( 114.0000000000000426, 15.53993994372673981, 7.305634244248866343E-16 ) ) ;
#11008=ORIENTED_EDGE ( 'NONE', *, *, #8157, .T. ) ;
#11018=LINE ( 'NONE', #13371, #878 ) ;
#11020=EDGE_CURVE ( 'NONE', #3704, #234, #3490, .T. ) ;
#11027=ORIENTED_EDGE ( 'NONE', *, *, #5991, .F. ) ;
#11029=DIRECTION ( 'NONE',  ( 0.000000000000000000, 0.000000000000000000, -1.000000000000000000 ) ) ;
#11031=DIRECTION ( 'NONE',  ( 0.000000000000000000, 0.9902680687415712502, 0.1391731009600586100 ) ) ;
#11033=EDGE_CURVE ( 'NONE', #5777, #13203, #12583, .T. ) ;
#11034=DIRECTION ( 'NONE',  ( 3.965082230804130220E-16, 4.956352788505162775E-17, -1.000000000000000000 ) ) ;
#11035=CARTESIAN_POINT ( 'NONE',  ( 184.0000000000000568, 15.53993994372673981, -12.49999999999999289 ) ) ;
#11038=FACE_OUTER_BOUND ( 'NONE', #8874, .T. ) ;
#11039=AXIS2_PLACEMENT_3D ( 'NONE', #3313, #6954, #9317 ) ;
#11042=LINE ( 'NONE', #10973, #5841 ) ;
#11043=AXIS2_PLACEMENT_3D ( 'NONE', #4259, #14417, #3539 ) ;
#11044=CARTESIAN_POINT ( 'NONE',  ( 190.0000000000000568, -178.8058001507315566, 52.19066787724494816 ) ) ;
#11045=CARTESIAN_POINT ( 'NONE',  ( 184.0000000000000568, -181.3058001507315566, 74.95141194869098911 ) ) ;
#11050=ORIENTED_EDGE ( 'NONE', *, *, #1187, .F. ) ;
#11053=EDGE_CURVE ( 'NONE', #720, #831, #14220, .T. ) ;
#11060=ADVANCED_FACE ( 'NONE', ( #5712 ), #9841, .T. ) ;
#11064=CARTESIAN_POINT ( 'NONE',  ( -63.50000000000002842, 17.53993994372673981, -17.50000000000002487 ) ) ;
#11065=LINE ( 'NONE', #217, #9862 ) ;
#11067=AXIS2_PLACEMENT_3D ( 'NONE', #171, #5019, #13213 ) ;
#11072=EDGE_CURVE ( 'NONE', #1807, #13446, #15602, .T. ) ;
#11074=CARTESIAN_POINT ( 'NONE',  ( 178.0000000000000853, 16.03993994372673981, 38.07518420361041933 ) ) ;
#11079=VECTOR ( 'NONE', #14628, 1000.000000000000000 ) ;
#11081=ORIENTED_EDGE ( 'NONE', *, *, #4214, .F. ) ;
#11086=DIRECTION ( 'NONE',  ( -1.000000000000000000, 0.000000000000000000, 0.000000000000000000 ) ) ;
#11088=CIRCLE ( 'NONE', #4257, 0.5000000000000004441 ) ;
#11089=DIRECTION ( 'NONE',  ( 0.000000000000000000, -0.1391731009600660485, -0.9902680687415702510 ) ) ;
#11090=AXIS2_PLACEMENT_3D ( 'NONE', #13278, #6274, #12106 ) ;
#11092=CARTESIAN_POINT ( 'NONE',  ( 178.0000000000000853, 15.17911304468680100, 9.062306170389884841 ) ) ;
#11093=AXIS2_PLACEMENT_3D ( 'NONE', #8039, #3367, #7005 ) ;
#11095=ORIENTED_EDGE ( 'NONE', *, *, #11728, .T. ) ;
#11096=DIRECTION ( 'NONE',  ( 1.000000000000000000, 2.751328491981765035E-32, -3.965082230804130220E-16 ) ) ;
#11100=VECTOR ( 'NONE', #8607, 1000.000000000000000 ) ;
#11102=ORIENTED_EDGE ( 'NONE', *, *, #2246, .T. ) ;
#11107=VERTEX_POINT ( 'NONE', #7607 ) ;
#11114=CARTESIAN_POINT ( 'NONE',  ( -63.50000000000002842, 15.60952649420677041, 9.122796835852554409 ) ) ;
#11126=FACE_OUTER_BOUND ( 'NONE', #8464, .T. ) ;
#11128=CARTESIAN_POINT ( 'NONE',  ( 177.5000000000000853, 15.03993994372673981, 10.05257423913146475 ) ) ;
#11130=CARTESIAN_POINT ( 'NONE',  ( 114.0000000000000426, 15.53993994372673981, 7.305634244248866343E-16 ) ) ;
#11139=ORIENTED_EDGE ( 'NONE', *, *, #3369, .T. ) ;
#11145=ORIENTED_EDGE ( 'NONE', *, *, #4111, .F. ) ;
#11146=DIRECTION ( 'NONE',  ( -1.000000000000000000, 0.000000000000000000, 0.000000000000000000 ) ) ;
#11148=TOROIDAL_SURFACE ( 'NONE', #7377, 1.000000000000000000, 0.5000000000000000000 ) ;
#11157=VERTEX_POINT ( 'NONE', #1271 ) ;
#11159=DIRECTION ( 'NONE',  ( -0.000000000000000000, -0.000000000000000000, 1.000000000000000000 ) ) ;
#11161=ORIENTED_EDGE ( 'NONE', *, *, #6028, .F. ) ;
#11164=ORIENTED_EDGE ( 'NONE', *, *, #13060, .F. ) ;
#11165=CARTESIAN_POINT ( 'NONE',  ( 190.5000000000000853, 15.60952649420676686, 25.87720316414728217 ) ) ;
#11169=EDGE_CURVE ( 'NONE', #552, #6305, #228, .T. ) ;
#11172=DIRECTION ( 'NONE',  ( -1.000000000000000000, 0.000000000000000000, 0.000000000000000000 ) ) ;
#11173=SURFACE_STYLE_USAGE ( .BOTH. , #7543 ) ;
#11179=DIRECTION ( 'NONE',  ( 1.504267769033196424E-15, -0.9902680687415713612, -0.1391731009600591373 ) ) ;
#11185=ORIENTED_EDGE ( 'NONE', *, *, #8664, .F. ) ;
#11188=DIRECTION ( 'NONE',  ( 0.000000000000000000, 0.000000000000000000, 1.000000000000000000 ) ) ;
#11189=DIRECTION ( 'NONE',  ( 0.000000000000000000, 1.000000000000000000, 6.938893903907227145E-17 ) ) ;
#11197=EDGE_CURVE ( 'NONE', #15235, #4643, #8198, .T. ) ;
#11208=AXIS2_PLACEMENT_3D ( 'NONE', #5454, #13647, #13892 ) ;
#11210=CARTESIAN_POINT ( 'NONE',  ( 184.0000000000000568, -201.3058001507315566, -41.45141194869120227 ) ) ;
#11211=CIRCLE ( 'NONE', #8454, 1.000000000000000888 ) ;
#11213=ADVANCED_FACE ( 'NONE', ( #11228 ), #14452, .F. ) ;
#11219=CARTESIAN_POINT ( 'NONE',  ( 190.0000000000000568, -178.8058001507315566, -30.31842631998718574 ) ) ;
#11220=EDGE_LOOP ( 'NONE', ( #13128, #11861, #13627, #8020 ) ) ;
#11221=DIRECTION ( 'NONE',  ( -1.000000000000000000, 0.000000000000000000, 3.965082230804112963E-16 ) ) ;
#11223=AXIS2_PLACEMENT_3D ( 'NONE', #12278, #1458, #8984 ) ;
#11224=DIRECTION ( 'NONE',  ( 0.000000000000000000, -0.000000000000000000, -1.000000000000000000 ) ) ;
#11228=FACE_OUTER_BOUND ( 'NONE', #2760, .T. ) ;
#11235=VERTEX_POINT ( 'NONE', #5677 ) ;
#11241=DIRECTION ( 'NONE',  ( 0.000000000000000000, 0.000000000000000000, 1.000000000000000000 ) ) ;
#11242=CARTESIAN_POINT ( 'NONE',  ( 190.0000000000000853, 14.90076684276667862, 37.08491613486884830 ) ) ;
#11243=CARTESIAN_POINT ( 'NONE',  ( -63.50000000000002842, -179.8058001507315566, -51.45141194869120227 ) ) ;
#11244=VECTOR ( 'NONE', #1823, 1000.000000000000114 ) ;
#11246=FILL_AREA_STYLE_COLOUR ( '', #8641 ) ;
#11256=EDGE_LOOP ( 'NONE', ( #8615, #1107, #3590, #15536 ) ) ;
#11257=EDGE_CURVE ( 'NONE', #8794, #12311, #15473, .T. ) ;
#11259=AXIS2_PLACEMENT_3D ( 'NONE', #5435, #4876, #13145 ) ;
#11263=CARTESIAN_POINT ( 'NONE',  ( 184.0000000000000568, -201.3058001507315566, 74.95141194869098911 ) ) ;
#11267=EDGE_CURVE ( 'NONE', #1631, #8808, #6788, .T. ) ;
#11269=FACE_OUTER_BOUND ( 'NONE', #9562, .T. ) ;
#11271=ORIENTED_EDGE ( 'NONE', *, *, #13957, .T. ) ;
#11273=ORIENTED_EDGE ( 'NONE', *, *, #11318, .F. ) ;
#11274=EDGE_LOOP ( 'NONE', ( #5731, #13844, #8041, #1709 ) ) ;
#11275=CARTESIAN_POINT ( 'NONE',  ( -63.50000000000002842, -179.8058001507315566, 52.19066787724494816 ) ) ;
#11276=CYLINDRICAL_SURFACE ( 'NONE', #4227, 0.5000000000000000000 ) ;
#11281=CARTESIAN_POINT ( 'NONE',  ( -76.00000000000001421, -179.3058001507315566, -30.31842631998718574 ) ) ;
#11292=AXIS2_PLACEMENT_3D ( 'NONE', #13237, #8228, #1240 ) ;
#11295=ORIENTED_EDGE ( 'NONE', *, *, #8976, .F. ) ;
#11296=VECTOR ( 'NONE', #2350, 1000.000000000000000 ) ;
#11301=ORIENTED_EDGE ( 'NONE', *, *, #14726, .T. ) ;
#11302=DIRECTION ( 'NONE',  ( 0.000000000000000000, -5.551115123125777653E-14, -1.000000000000000000 ) ) ;
#11303=VECTOR ( 'NONE', #12482, 1000.000000000000000 ) ;
#11307=CARTESIAN_POINT ( 'NONE',  ( -76.50000000000004263, 14.90076684276667507, 37.08491613486882699 ) ) ;
#11309=CIRCLE ( 'NONE', #8547, 0.5000000000000069944 ) ;
#11312=EDGE_CURVE ( 'NONE', #6346, #12639, #5748, .T. ) ;
#11315=LINE ( 'NONE', #5400, #14765 ) ;
#11316=CARTESIAN_POINT ( 'NONE',  ( -64.00000000000002842, 15.03993994372673981, 10.05257423913146475 ) ) ;
#11318=EDGE_CURVE ( 'NONE', #12158, #944, #11211, .T. ) ;
#11319=TOROIDAL_SURFACE ( 'NONE', #11822, 1.000000000000000000, 0.5000000000000000000 ) ;
#11323=FACE_OUTER_BOUND ( 'NONE', #7211, .T. ) ;
#11329=ORIENTED_EDGE ( 'NONE', *, *, #13348, .F. ) ;
#11332=CARTESIAN_POINT ( 'NONE',  ( -64.00000000000002842, 15.03993994372673981, 10.05257423913146475 ) ) ;
#11334=EDGE_CURVE ( 'NONE', #5911, #10463, #9698, .T. ) ;
#11344=VERTEX_POINT ( 'NONE', #6870 ) ;
#11345=CARTESIAN_POINT ( 'NONE',  ( 190.0000000000000568, 15.53993994372673804, 24.94742576086838781 ) ) ;
#11346=ORIENTED_EDGE ( 'NONE', *, *, #1567, .T. ) ;
#11347=ORIENTED_EDGE ( 'NONE', *, *, #13850, .T. ) ;
#11348=DIRECTION ( 'NONE',  ( 5.518327896226364679E-17, 0.9902680687415713612, -0.1391731009600582492 ) ) ;
#11351=DIRECTION ( 'NONE',  ( -0.000000000000000000, -0.000000000000000000, 1.000000000000000000 ) ) ;
#11360=VERTEX_POINT ( 'NONE', #11598 ) ;
#11361=FACE_OUTER_BOUND ( 'NONE', #11220, .T. ) ;
#11369=ORIENTED_EDGE ( 'NONE', *, *, #8346, .F. ) ;
#11375=DIRECTION ( 'NONE',  ( 0.000000000000000000, 0.000000000000000000, -1.000000000000000000 ) ) ;
#11379=DIRECTION ( 'NONE',  ( 0.000000000000000000, 0.000000000000000000, 1.000000000000000000 ) ) ;
#11380=EDGE_LOOP ( 'NONE', ( #3572, #9942, #4349, #6829 ) ) ;
#11383=DIRECTION ( 'NONE',  ( 2.751328491981765035E-32, 1.000000000000000000, 1.090924371466202084E-47 ) ) ;
#11384=ORIENTED_EDGE ( 'NONE', *, *, #4596, .F. ) ;
#11388=ORIENTED_EDGE ( 'NONE', *, *, #10607, .F. ) ;
#11389=ORIENTED_EDGE ( 'NONE', *, *, #4214, .T. ) ;
#11392=EDGE_CURVE ( 'NONE', #5020, #14786, #12765, .T. ) ;
#11396=LINE ( 'NONE', #11165, #7831 ) ;
#11397=CARTESIAN_POINT ( 'NONE',  ( -70.00000000000000000, 15.53993994372673626, 45.99999999999998579 ) ) ;
#11398=DIRECTION ( 'NONE',  ( 0.000000000000000000, 0.000000000000000000, -1.000000000000000000 ) ) ;
#11407=EDGE_CURVE ( 'NONE', #13191, #10895, #9957, .T. ) ;
#11413=LINE ( 'NONE', #7637, #6678 ) ;
#11415=ADVANCED_FACE ( 'NONE', ( #4881 ), #9623, .T. ) ;
#11441=DIRECTION ( 'NONE',  ( 0.000000000000000000, 0.000000000000000000, -1.000000000000000000 ) ) ;
#11444=CIRCLE ( 'NONE', #4123, 0.5000000000000004441 ) ;
#11448=ORIENTED_EDGE ( 'NONE', *, *, #13694, .F. ) ;
#11449=EDGE_CURVE ( 'NONE', #6079, #3829, #11830, .T. ) ;
#11451=DIRECTION ( 'NONE',  ( -1.000000000000000000, 0.000000000000000000, 0.000000000000000000 ) ) ;
#11452=AXIS2_PLACEMENT_3D ( 'NONE', #4212, #2816, #4064 ) ;
#11454=DIRECTION ( 'NONE',  ( 1.000000000000000000, -2.751328491981765035E-32, 3.965082230804130220E-16 ) ) ;
#11456=EDGE_CURVE ( 'NONE', #10340, #7288, #5906, .T. ) ;
#11466=LINE ( 'NONE', #14921, #11244 ) ;
#11467=ADVANCED_FACE ( 'NONE', ( #13305 ), #4956, .T. ) ;
#11472=DIRECTION ( 'NONE',  ( 0.000000000000000000, 0.1391731009600626345, 0.9902680687415706950 ) ) ;
#11473=FACE_OUTER_BOUND ( 'NONE', #3742, .T. ) ;
#11481=CARTESIAN_POINT ( 'NONE',  ( -64.00000000000002842, -179.3058001507315566, 84.88378295107887084 ) ) ;
#11482=ADVANCED_FACE ( 'NONE', ( #9464 ), #14263, .T. ) ;
#11483=CIRCLE ( 'NONE', #9220, 1.000000000000000888 ) ;
#11484=DIRECTION ( 'NONE',  ( 0.000000000000000000, 0.000000000000000000, -1.000000000000000000 ) ) ;
#11486=DIRECTION ( 'NONE',  ( -0.000000000000000000, 1.000000000000000000, -0.000000000000000000 ) ) ;
#11494=CARTESIAN_POINT ( 'NONE',  ( -63.50000000000002842, 15.03993994372673804, 24.94742576086838781 ) ) ;
#11503=CIRCLE ( 'NONE', #8985, 0.5000000000000004441 ) ;
#11505=CYLINDRICAL_SURFACE ( 'NONE', #7535, 0.5000000000000004441 ) ;
#11506=CARTESIAN_POINT ( 'NONE',  ( 177.5000000000000853, -181.3058001507315566, 84.88378295107885663 ) ) ;
#11507=ORIENTED_EDGE ( 'NONE', *, *, #10235, .T. ) ;
#11518=DIRECTION ( 'NONE',  ( 3.965082230804130220E-16, -4.956352788505162775E-17, 1.000000000000000000 ) ) ;
#11527=CARTESIAN_POINT ( 'NONE',  ( -76.50000000000001421, 16.03993994372673981, -17.50000000000002487 ) ) ;
#11537=VERTEX_POINT ( 'NONE', #345 ) ;
#11539=ORIENTED_EDGE ( 'NONE', *, *, #12964, .F. ) ;
#11540=ORIENTED_EDGE ( 'NONE', *, *, #12087, .F. ) ;
#11541=DIRECTION ( 'NONE',  ( -1.000000000000000000, 0.000000000000000000, 0.000000000000000000 ) ) ;
#11551=ADVANCED_FACE ( 'NONE', ( #13778 ), #14954, .T. ) ;
#11556=ORIENTED_EDGE ( 'NONE', *, *, #10311, .T. ) ;
#11558=AXIS2_PLACEMENT_3D ( 'NONE', #1857, #14013, #6700 ) ;
#11561=ORIENTED_EDGE ( 'NONE', *, *, #4940, .T. ) ;
#11564=ORIENTED_EDGE ( 'NONE', *, *, #10607, .T. ) ;
#11567=DIRECTION ( 'NONE',  ( -3.965082230804130220E-16, 4.956352788505162775E-17, -1.000000000000000000 ) ) ;
#11568=LINE ( 'NONE', #10156, #4673 ) ;
#11569=CARTESIAN_POINT ( 'NONE',  ( -63.50000000000002842, -179.3058001507315566, -51.45141194869120227 ) ) ;
#11570=CIRCLE ( 'NONE', #1481, 0.5000000000000004441 ) ;
#11573=ORIENTED_EDGE ( 'NONE', *, *, #8852, .F. ) ;
#11578=CARTESIAN_POINT ( 'NONE',  ( -63.50000000000002842, -179.3058001507315566, 84.88378295107887084 ) ) ;
#11579=ORIENTED_EDGE ( 'NONE', *, *, #6653, .F. ) ;
#11582=ORIENTED_EDGE ( 'NONE', *, *, #11267, .F. ) ;
#11589=CARTESIAN_POINT ( 'NONE',  ( -76.00000000000004263, 23.05038067821379499, 35.93956260393299829 ) ) ;
#11593=AXIS2_PLACEMENT_3D ( 'NONE', #7951, #15103, #13933 ) ;
#11598=CARTESIAN_POINT ( 'NONE',  ( 190.5000000000000568, -178.9449732516916072, -29.32815825124561471 ) ) ;
#11599=DIRECTION ( 'NONE',  ( 1.000000000000000000, 0.000000000000000000, 0.000000000000000000 ) ) ;
#11600=VECTOR ( 'NONE', #15348, 1000.000000000000000 ) ;
#11602=ORIENTED_EDGE ( 'NONE', *, *, #3824, .T. ) ;
#11603=CIRCLE ( 'NONE', #8834, 0.5000000000000004441 ) ;
#11604=CIRCLE ( 'NONE', #1501, 0.5000000000000004441 ) ;
#11606=ORIENTED_EDGE ( 'NONE', *, *, #7500, .T. ) ;
#11611=CARTESIAN_POINT ( 'NONE',  ( 190.0000000000000853, -179.3058001507315566, 52.19066787724494816 ) ) ;
#11612=LINE ( 'NONE', #1813, #1080 ) ;
#11614=VERTEX_POINT ( 'NONE', #8670 ) ;
#11618=EDGE_LOOP ( 'NONE', ( #14642, #14831, #12774, #15225 ) ) ;
#11621=DIRECTION ( 'NONE',  ( 1.000000000000000000, -0.000000000000000000, -0.000000000000000000 ) ) ;
#11625=CIRCLE ( 'NONE', #4816, 0.5000000000000004441 ) ;
#11627=ORIENTED_EDGE ( 'NONE', *, *, #7297, .F. ) ;
#11628=FACE_OUTER_BOUND ( 'NONE', #14522, .T. ) ;
#11629=DIRECTION ( 'NONE',  ( 0.000000000000000000, 0.000000000000000000, -1.000000000000000000 ) ) ;
#11633=FACE_OUTER_BOUND ( 'NONE', #2822, .T. ) ;
#11636=CARTESIAN_POINT ( 'NONE',  ( -64.00000000000002842, 16.03993994372673981, -3.075184203610571654 ) ) ;
#11637=LINE ( 'NONE', #11481, #13607 ) ;
#11645=ORIENTED_EDGE ( 'NONE', *, *, #14529, .F. ) ;
#11649=ADVANCED_FACE ( 'NONE', ( #3201 ), #15339, .F. ) ;
#11650=EDGE_CURVE ( 'NONE', #3571, #7716, #11980, .T. ) ;
#11654=CARTESIAN_POINT ( 'NONE',  ( -63.50000000000002842, -178.6666270497714777, -18.18093594598675011 ) ) ;
#11658=ORIENTED_EDGE ( 'NONE', *, *, #11650, .F. ) ;
#11659=CARTESIAN_POINT ( 'NONE',  ( -64.00000000000002842, 15.03993994372673804, 38.07518420361041933 ) ) ;
#11660=ORIENTED_EDGE ( 'NONE', *, *, #3369, .F. ) ;
#11672=FACE_OUTER_BOUND ( 'NONE', #12808, .T. ) ;
#11673=DIRECTION ( 'NONE',  ( 5.518327896226365911E-17, 0.9902680687415714722, -0.1391731009600582769 ) ) ;
#11680=EDGE_CURVE ( 'NONE', #4447, #7455, #15234, .T. ) ;
#11683=ORIENTED_EDGE ( 'NONE', *, *, #7328, .F. ) ;
#11687=AXIS2_PLACEMENT_3D ( 'NONE', #12924, #3218, #8140 ) ;
#11694=ORIENTED_EDGE ( 'NONE', *, *, #2540, .T. ) ;
#11695=EDGE_CURVE ( 'NONE', #5784, #9446, #6440, .T. ) ;
#11697=VERTEX_POINT ( 'NONE', #7885 ) ;
#11701=FACE_OUTER_BOUND ( 'NONE', #15054, .T. ) ;
#11702=CIRCLE ( 'NONE', #11452, 0.5000000000000004441 ) ;
#11703=PLANE ( 'NONE',  #9866 ) ;
#11708=CYLINDRICAL_SURFACE ( 'NONE', #1786, 0.5000000000000004441 ) ;
#11718=EDGE_LOOP ( 'NONE', ( #8715, #8435, #7091, #2333, #1020, #11388 ) ) ;
#11721=CYLINDRICAL_SURFACE ( 'NONE', #9066, 1.499999999999997780 ) ;
#11726=CARTESIAN_POINT ( 'NONE',  ( 177.5000000000000853, 17.53993994372673981, -17.50000000000002487 ) ) ;
#11728=EDGE_CURVE ( 'NONE', #11157, #10552, #5418, .T. ) ;
#11729=FACE_OUTER_BOUND ( 'NONE', #8538, .T. ) ;
#11732=EDGE_CURVE ( 'NONE', #11344, #10124, #3650, .T. ) ;
#11733=CARTESIAN_POINT ( 'NONE',  ( 178.0000000000000853, 15.10952649420676686, 25.44255979523916977 ) ) ;
#11739=DIRECTION ( 'NONE',  ( -1.000000000000000000, 0.000000000000000000, 0.000000000000000000 ) ) ;
#11742=DIRECTION ( 'NONE',  ( -3.965082230804130220E-16, -4.956352788505162775E-17, 1.000000000000000000 ) ) ;
#11753=ADVANCED_FACE ( 'NONE', ( #5583 ), #10391, .T. ) ;
#11755=DIRECTION ( 'NONE',  ( 1.000000000000000000, 0.000000000000000000, 0.000000000000000000 ) ) ;
#11757=DIRECTION ( 'NONE',  ( 0.000000000000000000, 4.956352788505162775E-17, -1.000000000000000000 ) ) ;
#11761=DIRECTION ( 'NONE',  ( 1.000000000000000000, -2.751328491981765035E-32, 3.965082230804130220E-16 ) ) ;
#11762=LINE ( 'NONE', #1165, #13905 ) ;
#11763=EDGE_LOOP ( 'NONE', ( #10692, #8889, #4666, #7909 ) ) ;
#11780=DIRECTION ( 'NONE',  ( 1.000000000000000000, 0.000000000000000000, 0.000000000000000000 ) ) ;
#11784=CARTESIAN_POINT ( 'NONE',  ( 178.0000000000000853, -178.6666270497714777, -18.18093594598673945 ) ) ;
#11787=ORIENTED_EDGE ( 'NONE', *, *, #8624, .T. ) ;
#11791=CARTESIAN_POINT ( 'NONE',  ( 190.5000000000000568, 14.97035339324670922, -2.580050169239785696 ) ) ;
#11801=CARTESIAN_POINT ( 'NONE',  ( -64.00000000000002842, -178.8753867012115961, -29.82329228561640022 ) ) ;
#11802=DIRECTION ( 'NONE',  ( -1.000000000000000000, 0.000000000000000000, 0.000000000000000000 ) ) ;
#11811=ORIENTED_EDGE ( 'NONE', *, *, #9302, .T. ) ;
#11816=LINE ( 'NONE', #4225, #7357 ) ;
#11819=ORIENTED_EDGE ( 'NONE', *, *, #6481, .T. ) ;
#11822=AXIS2_PLACEMENT_3D ( 'NONE', #9125, #571, #5409 ) ;
#11823=EDGE_CURVE ( 'NONE', #11943, #13871, #8956, .T. ) ;
#11825=DIRECTION ( 'NONE',  ( 0.000000000000000000, -0.000000000000000000, 1.000000000000000000 ) ) ;
#11827=LINE ( 'NONE', #13482, #8432 ) ;
#11828=DIRECTION ( 'NONE',  ( 1.000000000000000000, 0.000000000000000000, 0.000000000000000000 ) ) ;
#11829=VECTOR ( 'NONE', #15467, 1000.000000000000000 ) ;
#11830=LINE ( 'NONE', #4715, #1866 ) ;
#11845=EDGE_CURVE ( 'NONE', #12599, #12968, #14474, .T. ) ;
#11848=ORIENTED_EDGE ( 'NONE', *, *, #5953, .T. ) ;
#11849=VECTOR ( 'NONE', #12516, 1000.000000000000000 ) ;
#11850=ORIENTED_EDGE ( 'NONE', *, *, #11922, .T. ) ;
#11859=CARTESIAN_POINT ( 'NONE',  ( 184.0000000000000568, -179.3058001507315566, 77.95141194869098911 ) ) ;
#11861=ORIENTED_EDGE ( 'NONE', *, *, #12028, .T. ) ;
#11868=ORIENTED_EDGE ( 'NONE', *, *, #15474, .F. ) ;
#11870=VECTOR ( 'NONE', #15292, 1000.000000000000000 ) ;
#11873=AXIS2_PLACEMENT_3D ( 'NONE', #6304, #2017, #3133 ) ;
#11881=ORIENTED_EDGE ( 'NONE', *, *, #4730, .T. ) ;
#11886=AXIS2_PLACEMENT_3D ( 'NONE', #781, #8727, #12495 ) ;
#11896=ORIENTED_EDGE ( 'NONE', *, *, #8483, .T. ) ;
#11897=ORIENTED_EDGE ( 'NONE', *, *, #10794, .F. ) ;
#11899=LINE ( 'NONE', #9528, #9581 ) ;
#11900=EDGE_CURVE ( 'NONE', #9167, #8877, #3363, .T. ) ;
#11901=CARTESIAN_POINT ( 'NONE',  ( 190.5000000000000853, -178.6666270497714777, 53.18093594598651919 ) ) ;
#11902=PLANE ( 'NONE',  #387 ) ;
#11905=DIRECTION ( 'NONE',  ( 0.000000000000000000, 0.000000000000000000, -1.000000000000000000 ) ) ;
#11908=EDGE_CURVE ( 'NONE', #10751, #14668, #11483, .T. ) ;
#11911=FACE_OUTER_BOUND ( 'NONE', #10222, .T. ) ;
#11912=ORIENTED_EDGE ( 'NONE', *, *, #4226, .T. ) ;
#11920=CLOSED_SHELL ( 'NONE', ( #13102, #6801, #4704, #14904, #3691, #691, #10116, #12724, #2116, #8563, #15434, #7326, #9160, #4397, #14198, #2968, #1506, #365, #15055, #1041, #2842, #2820, #13540, #6053, #15490, #5203, #8134, #13623, #4958, #9357, #607, #14984, #5275, #2019, #3211, #8515, #7287, #10715, #8195, #7478, #14759, #5868, #8383, #190, #13745, #3725, #12002, #4991, #2111, #6497, #10158, #9789, #9439, #5347, #12588, #934, #5933, #1399, #14823, #4336, #11060, #7101, #6246, #7160, #9259, #676, #5115, #10941, #9972, #14278, #6376, #11753, #5130, #13464, #11649, #8992 ) ) ;
#11921=DIRECTION ( 'NONE',  ( 0.000000000000000000, 1.000000000000000000, 6.938893903907227145E-17 ) ) ;
#11922=EDGE_CURVE ( 'NONE', #1631, #552, #5966, .T. ) ;
#11925=VERTEX_POINT ( 'NONE', #12038 ) ;
#11926=EDGE_CURVE ( 'NONE', #7344, #6077, #3515, .T. ) ;
#11928=CARTESIAN_POINT ( 'NONE',  ( -76.50000000000001421, -179.8058001507315566, -51.45141194869120227 ) ) ;
#11943=VERTEX_POINT ( 'NONE', #8503 ) ;
#11944=EDGE_CURVE ( 'NONE', #3832, #2866, #8352, .T. ) ;
#11948=LINE ( 'NONE', #12170, #9533 ) ;
#11950=DIRECTION ( 'NONE',  ( 0.000000000000000000, 0.000000000000000000, -1.000000000000000000 ) ) ;
#11953=ORIENTED_EDGE ( 'NONE', *, *, #8671, .F. ) ;
#11954=ORIENTED_EDGE ( 'NONE', *, *, #6481, .F. ) ;
#11960=DIRECTION ( 'NONE',  ( 0.000000000000000000, -1.000000000000000000, 0.000000000000000000 ) ) ;
#11961=CARTESIAN_POINT ( 'NONE',  ( -70.00000000000000000, -181.3058001507315566, 76.45141194869098911 ) ) ;
#11979=FACE_OUTER_BOUND ( 'NONE', #6740, .T. ) ;
#11980=CIRCLE ( 'NONE', #2643, 1.499999999999994449 ) ;
#11984=CARTESIAN_POINT ( 'NONE',  ( -70.00000000000000000, -201.3058001507315566, 76.45141194869098911 ) ) ;
#11990=CARTESIAN_POINT ( 'NONE',  ( -64.00000000000002842, 11.87216911405866959, 26.40245448993442068 ) ) ;
#11993=EDGE_LOOP ( 'NONE', ( #10150, #12708, #5625, #12917 ) ) ;
#11994=DIRECTION ( 'NONE',  ( 0.000000000000000000, 0.000000000000000000, -1.000000000000000000 ) ) ;
#12001=CIRCLE ( 'NONE', #1384, 1.000000000000000888 ) ;
#12002=ADVANCED_FACE ( 'NONE', ( #11323 ), #14706, .T. ) ;
#12008=ORIENTED_EDGE ( 'NONE', *, *, #9467, .F. ) ;
#12010=ORIENTED_EDGE ( 'NONE', *, *, #14429, .T. ) ;
#12011=EDGE_LOOP ( 'NONE', ( #8400, #2847, #8922, #10655 ) ) ;
#12012=LINE ( 'NONE', #12082, #6021 ) ;
#12014=VERTEX_POINT ( 'NONE', #8577 ) ;
#12015=CARTESIAN_POINT ( 'NONE',  ( 190.0000000000000568, 15.10952649420676863, 9.557440204760682789 ) ) ;
#12016=EDGE_CURVE ( 'NONE', #4972, #4326, #11018, .T. ) ;
#12019=VERTEX_POINT ( 'NONE', #168 ) ;
#12028=EDGE_CURVE ( 'NONE', #85, #14199, #8653, .T. ) ;
#12029=ADVANCED_FACE ( 'NONE', ( #14070, #15244 ), #13924, .T. ) ;
#12038=CARTESIAN_POINT ( 'NONE',  ( -76.50000000000001421, 15.03993994372673981, -2.075184203610571210 ) ) ;
#12040=DIRECTION ( 'NONE',  ( -3.965082230804130220E-16, -4.956352788505162775E-17, 1.000000000000000000 ) ) ;
#12041=EDGE_LOOP ( 'NONE', ( #9513, #14227, #4590, #7520 ) ) ;
#12050=CARTESIAN_POINT ( 'NONE',  ( -64.00000000000002842, 15.03993994372673804, 38.07518420361041933 ) ) ;
#12055=DIRECTION ( 'NONE',  ( 0.000000000000000000, -1.734723475976808672E-15, 1.000000000000000000 ) ) ;
#12059=CARTESIAN_POINT ( 'NONE',  ( 114.0000000000000426, 17.53993994372673981, 8.693413025030312018E-16 ) ) ;
#12060=VERTEX_POINT ( 'NONE', #1008 ) ;
#12067=CARTESIAN_POINT ( 'NONE',  ( 177.5000000000000853, -181.3058001507315566, -51.45141194869119516 ) ) ;
#12070=DIRECTION ( 'NONE',  ( -0.000000000000000000, 1.000000000000000000, -0.000000000000000000 ) ) ;
#12071=CYLINDRICAL_SURFACE ( 'NONE', #185, 0.5000000000000004441 ) ;
#12072=EDGE_LOOP ( 'NONE', ( #5814, #2594, #4785, #2651 ) ) ;
#12073=AXIS2_PLACEMENT_3D ( 'NONE', #10536, #15332, #894 ) ;
#12074=TOROIDAL_SURFACE ( 'NONE', #15333, 1.000000000000000000, 0.5000000000000000000 ) ;
#12077=VERTEX_POINT ( 'NONE', #9123 ) ;
#12078=AXIS2_PLACEMENT_3D ( 'NONE', #2239, #1284, #13 ) ;
#12081=VERTEX_POINT ( 'NONE', #5563 ) ;
#12082=CARTESIAN_POINT ( 'NONE',  ( 177.5000000000000853, -179.2362136002515740, 53.26098611522623827 ) ) ;
#12083=FACE_OUTER_BOUND ( 'NONE', #15384, .T. ) ;
#12086=LINE ( 'NONE', #1264, #480 ) ;
#12087=EDGE_CURVE ( 'NONE', #6953, #3135, #12652, .T. ) ;
#12088=AXIS2_PLACEMENT_3D ( 'NONE', #12413, #558, #396 ) ;
#12095=CARTESIAN_POINT ( 'NONE',  ( 177.5000000000000853, -178.8058001507315566, 65.31842631998698323 ) ) ;
#12096=EDGE_CURVE ( 'NONE', #592, #3561, #13762, .T. ) ;
#12105=DIRECTION ( 'NONE',  ( 1.077120774387149835E-15, 0.9902680687415711391, -0.1391731009600592484 ) ) ;
#12106=DIRECTION ( 'NONE',  ( 0.000000000000000000, -0.1391731009600592484, -0.9902680687415712502 ) ) ;
#12110=AXIS2_PLACEMENT_3D ( 'NONE', #2819, #7641, #12433 ) ;
#12111=( NAMED_UNIT ( * ) PLANE_ANGLE_UNIT ( ) SI_UNIT ( $, .RADIAN. ) );
#12117=CARTESIAN_POINT ( 'NONE',  ( 178.0000000000000853, -178.8058001507315566, -18.19066787724516843 ) ) ;
#12131=LINE ( 'NONE', #15511, #1913 ) ;
#12134=AXIS2_PLACEMENT_3D ( 'NONE', #3544, #8378, #13160 ) ;
#12140=VERTEX_POINT ( 'NONE', #7783 ) ;
#12141=ORIENTED_EDGE ( 'NONE', *, *, #3635, .F. ) ;
#12143=DIRECTION ( 'NONE',  ( 0.000000000000000000, 4.956352788505162775E-17, -1.000000000000000000 ) ) ;
#12144=FACE_OUTER_BOUND ( 'NONE', #13103, .T. ) ;
#12145=EDGE_CURVE ( 'NONE', #11235, #11925, #13229, .T. ) ;
#12146=CARTESIAN_POINT ( 'NONE',  ( 190.0000000000000568, -178.8058001507315566, 52.19066787724494816 ) ) ;
#12151=ORIENTED_EDGE ( 'NONE', *, *, #11823, .F. ) ;
#12158=VERTEX_POINT ( 'NONE', #6682 ) ;
#12163=CARTESIAN_POINT ( 'NONE',  ( 190.0000000000000568, 14.90076684276668040, -2.084916134869001958 ) ) ;
#12164=DIRECTION ( 'NONE',  ( 1.000000000000000000, -0.000000000000000000, -0.000000000000000000 ) ) ;
#12167=CIRCLE ( 'NONE', #10923, 1.499999999999997780 ) ;
#12168=ORIENTED_EDGE ( 'NONE', *, *, #4052, .F. ) ;
#12170=CARTESIAN_POINT ( 'NONE',  ( 190.5000000000000853, -179.8058001507315566, 84.88378295107887084 ) ) ;
#12171=ORIENTED_EDGE ( 'NONE', *, *, #9853, .T. ) ;
#12173=CARTESIAN_POINT ( 'NONE',  ( -63.50000000000002842, -179.2362136002515740, 53.26098611522623827 ) ) ;
#12174=CARTESIAN_POINT ( 'NONE',  ( -76.00000000000004263, -178.8753867012115961, 64.82329228561619061 ) ) ;
#12183=CARTESIAN_POINT ( 'NONE',  ( -63.50000000000002842, 16.03993994372673981, 25.38206912977649665 ) ) ;
#12187=VERTEX_POINT ( 'NONE', #13114 ) ;
#12188=DIRECTION ( 'NONE',  ( 0.000000000000000000, 0.000000000000000000, -1.000000000000000000 ) ) ;
#12191=FACE_OUTER_BOUND ( 'NONE', #12011, .T. ) ;
#12192=ORIENTED_EDGE ( 'NONE', *, *, #6928, .F. ) ;
#12200=DIRECTION ( 'NONE',  ( 0.000000000000000000, 0.000000000000000000, 1.000000000000000000 ) ) ;
#12201=CARTESIAN_POINT ( 'NONE',  ( 175.9483885134608272, -178.8058001507315566, -17.19066787724516843 ) ) ;
#12202=FACE_OUTER_BOUND ( 'NONE', #12832, .T. ) ;
#12203=VECTOR ( 'NONE', #14834, 1000.000000000000000 ) ;
#12205=EDGE_CURVE ( 'NONE', #8310, #14585, #4843, .T. ) ;
#12208=EDGE_CURVE ( 'NONE', #1178, #14048, #4414, .T. ) ;
#12211=PLANE ( 'NONE',  #12805 ) ;
#12213=ORIENTED_EDGE ( 'NONE', *, *, #3994, .F. ) ;
#12217=DIRECTION ( 'NONE',  ( 0.000000000000000000, 0.000000000000000000, -1.000000000000000000 ) ) ;
#12218=CARTESIAN_POINT ( 'NONE',  ( -64.00000000000002842, 15.53993994372673804, 37.49999999999991473 ) ) ;
#12219=CARTESIAN_POINT ( 'NONE',  ( 190.5000000000000568, 15.03993994372673981, 10.05257423913146475 ) ) ;
#12223=CARTESIAN_POINT ( 'NONE',  ( -76.00000000000004263, 15.10952649420676686, 25.44255979523916977 ) ) ;
#12225=EDGE_CURVE ( 'NONE', #944, #12081, #9979, .T. ) ;
#12227=ORIENTED_EDGE ( 'NONE', *, *, #455, .T. ) ;
#12228=VECTOR ( 'NONE', #2409, 1000.000000000000000 ) ;
#12241=EDGE_LOOP ( 'NONE', ( #14435, #11507, #4962, #10513 ) ) ;
#12244=ORIENTED_EDGE ( 'NONE', *, *, #4319, .T. ) ;
#12246=ORIENTED_EDGE ( 'NONE', *, *, #2352, .F. ) ;
#12247=LINE ( 'NONE', #12173, #7220 ) ;
#12248=ADVANCED_FACE ( 'NONE', ( #13029 ), #7226, .F. ) ;
#12250=ORIENTED_EDGE ( 'NONE', *, *, #445, .F. ) ;
#12251=ORIENTED_EDGE ( 'NONE', *, *, #2572, .T. ) ;
#12260=EDGE_CURVE ( 'NONE', #8201, #5020, #2152, .T. ) ;
#12262=ORIENTED_EDGE ( 'NONE', *, *, #225, .F. ) ;
#12268=EDGE_CURVE ( 'NONE', #14171, #8310, #14296, .T. ) ;
#12271=ORIENTED_EDGE ( 'NONE', *, *, #3338, .F. ) ;
#12273=CARTESIAN_POINT ( 'NONE',  ( -63.50000000000002842, -178.8058001507315566, 52.19066787724494816 ) ) ;
#12276=CARTESIAN_POINT ( 'NONE',  ( 190.5000000000000568, 17.53993994372673981, -17.50000000000002487 ) ) ;
#12278=CARTESIAN_POINT ( 'NONE',  ( -64.00000000000002842, -179.8058001507315566, 52.49999999999997868 ) ) ;
#12282=ORIENTED_EDGE ( 'NONE', *, *, #7340, .T. ) ;
#12286=ORIENTED_EDGE ( 'NONE', *, *, #13550, .T. ) ;
#12287=DIRECTION ( 'NONE',  ( -0.000000000000000000, -0.9902680687415712502, -0.1391731009600584990 ) ) ;
#12290=AXIS2_PLACEMENT_3D ( 'NONE', #14182, #5905, #2270 ) ;
#12293=LINE ( 'NONE', #13714, #9257 ) ;
#12294=DIRECTION ( 'NONE',  ( 0.000000000000000000, 0.000000000000000000, 1.000000000000000000 ) ) ;
#12296=EDGE_LOOP ( 'NONE', ( #2575, #7833, #5004, #9965 ) ) ;
#12304=EDGE_CURVE ( 'NONE', #2049, #14442, #10849, .T. ) ;
#12306=EDGE_CURVE ( 'NONE', #4671, #7084, #13490, .T. ) ;
#12308=VERTEX_POINT ( 'NONE', #9739 ) ;
#12311=VERTEX_POINT ( 'NONE', #7379 ) ;
#12313=CARTESIAN_POINT ( 'NONE',  ( 177.5000000000000853, 15.17911304468680100, 9.062306170389884841 ) ) ;
#12317=FACE_BOUND ( 'NONE', #5790, .T. ) ;
#12318=ORIENTED_EDGE ( 'NONE', *, *, #915, .T. ) ;
#12322=CIRCLE ( 'NONE', #5025, 0.5000000000000000000 ) ;
#12325=DIRECTION ( 'NONE',  ( 1.000000000000000000, -2.751328491981765035E-32, 3.965082230804130220E-16 ) ) ;
#12326=AXIS2_PLACEMENT_3D ( 'NONE', #2810, #7631, #1615 ) ;
#12332=ORIENTED_EDGE ( 'NONE', *, *, #13260, .F. ) ;
#12333=FACE_OUTER_BOUND ( 'NONE', #5177, .T. ) ;
#12335=AXIS2_PLACEMENT_3D ( 'NONE', #5235, #1600, #11086 ) ;
#12336=DIRECTION ( 'NONE',  ( 0.000000000000000000, -6.938893903907222067E-15, 1.000000000000000000 ) ) ;
#12337=AXIS2_PLACEMENT_3D ( 'NONE', #4568, #8147, #5681 ) ;
#12339=DIRECTION ( 'NONE',  ( 0.000000000000000000, 4.956352788505162775E-17, -1.000000000000000000 ) ) ;
#12348=CARTESIAN_POINT ( 'NONE',  ( -76.00000000000001421, 14.97035339324670922, -2.580050169239785696 ) ) ;
#12358=CYLINDRICAL_SURFACE ( 'NONE', #6580, 0.5000000000000004441 ) ;
#12362=PLANE ( 'NONE',  #1852 ) ;
#12365=AXIS2_PLACEMENT_3D ( 'NONE', #13893, #9093, #3088 ) ;
#12367=EDGE_LOOP ( 'NONE', ( #3418, #1193, #14441, #7526 ) ) ;
#12371=VERTEX_POINT ( 'NONE', #9978 ) ;
#12373=CARTESIAN_POINT ( 'NONE',  ( 190.5000000000000853, -179.8058001507315566, 65.31842631998698323 ) ) ;
#12376=DIRECTION ( 'NONE',  ( -3.965082230804130220E-16, -4.956352788505162775E-17, 1.000000000000000000 ) ) ;
#12382=CYLINDRICAL_SURFACE ( 'NONE', #7921, 1.499999999999994449 ) ;
#12383=CIRCLE ( 'NONE', #1543, 0.5000000000000004441 ) ;
#12386=EDGE_LOOP ( 'NONE', ( #6874, #9981, #8390, #5058 ) ) ;
#12388=ORIENTED_EDGE ( 'NONE', *, *, #8657, .T. ) ;
#12395=ADVANCED_FACE ( 'NONE', ( #7611, #8783 ), #14838, .T. ) ;
#12396=DIRECTION ( 'NONE',  ( 0.000000000000000000, -1.000000000000000000, -6.938893903907227145E-17 ) ) ;
#12398=EDGE_CURVE ( 'NONE', #8073, #427, #12247, .T. ) ;
#12400=CIRCLE ( 'NONE', #13654, 0.5000000000000004441 ) ;
#12405=VERTEX_POINT ( 'NONE', #6188 ) ;
#12406=DIRECTION ( 'NONE',  ( 0.000000000000000000, -1.000000000000000000, -4.956352788505162775E-17 ) ) ;
#12407=FACE_BOUND ( 'NONE', #7766, .T. ) ;
#12413=CARTESIAN_POINT ( 'NONE',  ( -70.00000000000000000, 17.53993994372673626, 47.49999999999997868 ) ) ;
#12415=FACE_OUTER_BOUND ( 'NONE', #4902, .T. ) ;
#12424=EDGE_LOOP ( 'NONE', ( #9390, #1826 ) ) ;
#12428=ORIENTED_EDGE ( 'NONE', *, *, #7640, .T. ) ;
#12432=FACE_BOUND ( 'NONE', #3043, .T. ) ;
#12433=DIRECTION ( 'NONE',  ( 0.000000000000000000, 0.000000000000000000, 1.000000000000000000 ) ) ;
#12446=EDGE_CURVE ( 'NONE', #2049, #9261, #4160, .T. ) ;
#12448=LINE ( 'NONE', #1637, #3007 ) ;
#12453=DIRECTION ( 'NONE',  ( 0.000000000000000000, -0.1391731009600641333, -0.9902680687415704730 ) ) ;
#12456=AXIS2_PLACEMENT_3D ( 'NONE', #8068, #8231, #2043 ) ;
#12458=FACE_OUTER_BOUND ( 'NONE', #1763, .T. ) ;
#12460=DIRECTION ( 'NONE',  ( -1.000000000000000000, 0.000000000000000000, 0.000000000000000000 ) ) ;
#12463=ORIENTED_EDGE ( 'NONE', *, *, #3894, .F. ) ;
#12467=DIRECTION ( 'NONE',  ( -0.000000000000000000, -1.000000000000000000, -6.938893903907227145E-17 ) ) ;
#12469=EDGE_CURVE ( 'NONE', #10853, #8326, #5936, .T. ) ;
#12474=DIRECTION ( 'NONE',  ( 0.000000000000000000, 0.000000000000000000, 1.000000000000000000 ) ) ;
#12480=ORIENTED_EDGE ( 'NONE', *, *, #4482, .T. ) ;
#12481=ORIENTED_EDGE ( 'NONE', *, *, #5985, .T. ) ;
#12482=DIRECTION ( 'NONE',  ( 0.000000000000000000, 0.000000000000000000, -1.000000000000000000 ) ) ;
#12485=ORIENTED_EDGE ( 'NONE', *, *, #14295, .T. ) ;
#12486=DIRECTION ( 'NONE',  ( 1.000000000000000000, -2.751328491981765035E-32, 3.965082230804130220E-16 ) ) ;
#12488=CARTESIAN_POINT ( 'NONE',  ( -76.00000000000004263, 15.53993994372673626, 52.49999999999997868 ) ) ;
#12492=AXIS2_PLACEMENT_3D ( 'NONE', #7878, #10310, #1774 ) ;
#12495=DIRECTION ( 'NONE',  ( 0.000000000000000000, 0.000000000000000000, -1.000000000000000000 ) ) ;
#12498=DIRECTION ( 'NONE',  ( -0.000000000000000000, 0.9902680687415713612, -0.1391731009600582492 ) ) ;
#12503=EDGE_LOOP ( 'NONE', ( #4829, #11683, #7610, #3885, #1348, #4519, #2318, #12481, #615 ) ) ;
#12508=FACE_OUTER_BOUND ( 'NONE', #5695, .T. ) ;
#12510=CARTESIAN_POINT ( 'NONE',  ( -76.50000000000001421, -181.3058001507315566, 84.88378295107885663 ) ) ;
#12515=DIRECTION ( 'NONE',  ( 1.000000000000000000, 0.000000000000000000, 0.000000000000000000 ) ) ;
#12516=DIRECTION ( 'NONE',  ( -0.000000000000000000, 0.000000000000000000, 1.000000000000000000 ) ) ;
#12520=EDGE_LOOP ( 'NONE', ( #5202, #4245, #8662, #7614 ) ) ;
#12521=LINE ( 'NONE', #7574, #14583 ) ;
#12522=DIRECTION ( 'NONE',  ( -0.000000000000000000, 0.000000000000000000, 1.000000000000000000 ) ) ;
#12530=DIRECTION ( 'NONE',  ( -3.965082230804130220E-16, -0.000000000000000000, -1.000000000000000000 ) ) ;
#12532=ORIENTED_EDGE ( 'NONE', *, *, #8157, .F. ) ;
#12533=CIRCLE ( 'NONE', #7521, 0.5000000000000004441 ) ;
#12538=VERTEX_POINT ( 'NONE', #5386 ) ;
#12542=AXIS2_PLACEMENT_3D ( 'NONE', #2200, #7032, #1558 ) ;
#12544=ORIENTED_EDGE ( 'NONE', *, *, #6535, .F. ) ;
#12552=CARTESIAN_POINT ( 'NONE',  ( -64.00000000000002842, -179.3058001507315566, 65.31842631998698323 ) ) ;
#12556=DIRECTION ( 'NONE',  ( 0.000000000000000000, 0.000000000000000000, -1.000000000000000000 ) ) ;
#12563=DIRECTION ( 'NONE',  ( 0.000000000000000000, 0.000000000000000000, 1.000000000000000000 ) ) ;
#12565=AXIS2_PLACEMENT_3D ( 'NONE', #6155, #8377, #3464 ) ;
#12566=ADVANCED_FACE ( 'NONE', ( #10207, #699, #3018 ), #4347, .T. ) ;
#12569=CARTESIAN_POINT ( 'NONE',  ( -76.50000000000001421, -178.7362136002515172, -17.68580191161595394 ) ) ;
#12571=CARTESIAN_POINT ( 'NONE',  ( -64.00000000000002842, -179.8058001507315566, 52.19066787724494816 ) ) ;
#12572=ORIENTED_EDGE ( 'NONE', *, *, #537, .F. ) ;
#12576=CIRCLE ( 'NONE', #12078, 0.5000000000000001110 ) ;
#12577=AXIS2_PLACEMENT_3D ( 'NONE', #8951, #3099, #5153 ) ;
#12583=CIRCLE ( 'NONE', #15353, 0.5000000000000004441 ) ;
#12584=CIRCLE ( 'NONE', #5796, 1.499999999999997780 ) ;
#12586=PRODUCT_DEFINITION ( 'UNKNOWN', '', #2745, #15279 ) ;
#12587=EDGE_CURVE ( 'NONE', #7467, #12158, #12001, .T. ) ;
#12588=ADVANCED_FACE ( 'NONE', ( #6737 ), #890, .T. ) ;
#12589=VERTEX_POINT ( 'NONE', #1973 ) ;
#12593=FACE_OUTER_BOUND ( 'NONE', #4353, .T. ) ;
#12594=EDGE_CURVE ( 'NONE', #12968, #1955, #7849, .T. ) ;
#12597=LINE ( 'NONE', #5346, #3553 ) ;
#12599=VERTEX_POINT ( 'NONE', #783 ) ;
#12600=AXIS2_PLACEMENT_3D ( 'NONE', #9345, #10602, #9416 ) ;
#12602=CARTESIAN_POINT ( 'NONE',  ( 175.9483885134608272, -179.3058001507315566, 84.88378295107887084 ) ) ;
#12607=DIRECTION ( 'NONE',  ( 1.000000000000000000, -2.751328491981765035E-32, 3.965082230804130220E-16 ) ) ;
#12609=LINE ( 'NONE', #15045, #4684 ) ;
#12610=EDGE_CURVE ( 'NONE', #12371, #12789, #9476, .T. ) ;
#12621=ORIENTED_EDGE ( 'NONE', *, *, #1267, .T. ) ;
#12624=ORIENTED_EDGE ( 'NONE', *, *, #12225, .F. ) ;
#12628=EDGE_CURVE ( 'NONE', #14434, #7029, #11466, .T. ) ;
#12629=CIRCLE ( 'NONE', #800, 0.9999999999999991118 ) ;
#12636=CARTESIAN_POINT ( 'NONE',  ( 190.0000000000000568, 15.53993994372674159, 9.617930870223352358 ) ) ;
#12639=VERTEX_POINT ( 'NONE', #8950 ) ;
#12641=VECTOR ( 'NONE', #6808, 1000.000000000000000 ) ;
#12647=FACE_OUTER_BOUND ( 'NONE', #5845, .T. ) ;
#12652=LINE ( 'NONE', #4130, #10220 ) ;
#12654=CARTESIAN_POINT ( 'NONE',  ( 190.0000000000000568, 15.03993994372673981, -3.075184203610571654 ) ) ;
#12658=VERTEX_POINT ( 'NONE', #12552 ) ;
#12666=VERTEX_POINT ( 'NONE', #628 ) ;
#12671=VERTEX_POINT ( 'NONE', #5768 ) ;
#12672=ADVANCED_FACE ( 'NONE', ( #4499 ), #10748, .F. ) ;
#12673=AXIS2_PLACEMENT_3D ( 'NONE', #4811, #9631, #8527 ) ;
#12688=DIRECTION ( 'NONE',  ( -0.000000000000000000, 0.9902680687415712502, 0.1391731009600586100 ) ) ;
#12689=CARTESIAN_POINT ( 'NONE',  ( -63.50000000000002842, 16.03993994372673981, 24.94742576086838781 ) ) ;
#12692=AXIS2_PLACEMENT_3D ( 'NONE', #1156, #6145, #3380 ) ;
#12694=DIRECTION ( 'NONE',  ( 0.000000000000000000, 0.000000000000000000, -1.000000000000000000 ) ) ;
#12697=VECTOR ( 'NONE', #3982, 1000.000000000000000 ) ;
#12700=CARTESIAN_POINT ( 'NONE',  ( -63.50000000000002842, -179.8058001507315566, -30.31842631998718574 ) ) ;
#12701=DIRECTION ( 'NONE',  ( 3.965082230804130220E-16, 4.956352788505162775E-17, -1.000000000000000000 ) ) ;
#12707=PLANE ( 'NONE',  #10812 ) ;
#12708=ORIENTED_EDGE ( 'NONE', *, *, #15572, .T. ) ;
#12711=DIRECTION ( 'NONE',  ( 1.000000000000000000, 0.000000000000000000, 0.000000000000000000 ) ) ;
#12712=ORIENTED_EDGE ( 'NONE', *, *, #15474, .T. ) ;
#12713=ORIENTED_EDGE ( 'NONE', *, *, #2003, .F. ) ;
#12724=ADVANCED_FACE ( 'NONE', ( #11701 ), #9733, .T. ) ;
#12725=EDGE_CURVE ( 'NONE', #2355, #13002, #6959, .T. ) ;
#12730=ORIENTED_EDGE ( 'NONE', *, *, #14936, .T. ) ;
#12736=AXIS2_PLACEMENT_3D ( 'NONE', #3345, #8181, #12962 ) ;
#12738=FACE_OUTER_BOUND ( 'NONE', #9067, .T. ) ;
#12739=VECTOR ( 'NONE', #6823, 1000.000000000000000 ) ;
#12748=DIRECTION ( 'NONE',  ( 0.000000000000000000, 1.000000000000000000, 6.938893903907227145E-17 ) ) ;
#12750=VERTEX_POINT ( 'NONE', #5852 ) ;
#12751=VECTOR ( 'NONE', #14063, 1000.000000000000000 ) ;
#12752=DIRECTION ( 'NONE',  ( 3.965082230804130220E-16, 1.090924371466202084E-47, 1.000000000000000000 ) ) ;
#12754=ORIENTED_EDGE ( 'NONE', *, *, #11072, .T. ) ;
#12756=DIRECTION ( 'NONE',  ( 0.000000000000000000, -0.000000000000000000, 1.000000000000000000 ) ) ;
#12760=CARTESIAN_POINT ( 'NONE',  ( -63.50000000000002842, 16.03993994372673981, -2.500000000000071498 ) ) ;
#12763=FACE_OUTER_BOUND ( 'NONE', #7918, .T. ) ;
#12764=CARTESIAN_POINT ( 'NONE',  ( -64.00000000000002842, -178.8058001507315566, -17.69066787724516843 ) ) ;
#12765=LINE ( 'NONE', #15594, #8942 ) ;
#12767=LINE ( 'NONE', #10568, #15121 ) ;
#12771=ORIENTED_EDGE ( 'NONE', *, *, #4196, .T. ) ;
#12773=DIRECTION ( 'NONE',  ( 1.000000000000000000, 0.000000000000000000, 0.000000000000000000 ) ) ;
#12774=ORIENTED_EDGE ( 'NONE', *, *, #3635, .T. ) ;
#12777=DIRECTION ( 'NONE',  ( -0.000000000000000000, 1.000000000000000000, -0.000000000000000000 ) ) ;
#12780=EDGE_CURVE ( 'NONE', #15235, #2394, #13756, .T. ) ;
#12782=EDGE_CURVE ( 'NONE', #7029, #4447, #7902, .T. ) ;
#12784=DIRECTION ( 'NONE',  ( -1.000000000000000000, 0.000000000000000000, 0.000000000000000000 ) ) ;
#12788=EDGE_LOOP ( 'NONE', ( #12480, #2343, #1515, #6237 ) ) ;
#12789=VERTEX_POINT ( 'NONE', #1870 ) ;
#12795=CARTESIAN_POINT ( 'NONE',  ( -63.50000000000002842, 15.03993994372673804, 37.07518420361041933 ) ) ;
#12797=CARTESIAN_POINT ( 'NONE',  ( 175.9483885134608272, -178.8058001507315566, 52.19066787724494816 ) ) ;
#12798=LINE ( 'NONE', #10218, #4436 ) ;
#12804=DIRECTION ( 'NONE',  ( 0.000000000000000000, 1.000000000000000000, 0.000000000000000000 ) ) ;
#12805=AXIS2_PLACEMENT_3D ( 'NONE', #347, #2668, #7486 ) ;
#12807=CARTESIAN_POINT ( 'NONE',  ( 175.9483885134608272, 15.53993994372673981, 37.49999999999991473 ) ) ;
#12808=EDGE_LOOP ( 'NONE', ( #4133, #10478, #8575, #3086, #15581, #6582 ) ) ;
#12812=VERTEX_POINT ( 'NONE', #602 ) ;
#12814=CARTESIAN_POINT ( 'NONE',  ( -76.50000000000001421, 14.90076684276668040, -2.084916134869001958 ) ) ;
#12815=CARTESIAN_POINT ( 'NONE',  ( -76.00000000000004263, 15.53993994372673804, 37.49999999999991473 ) ) ;
#12826=CIRCLE ( 'NONE', #12335, 0.5000000000000004441 ) ;
#12829=ORIENTED_EDGE ( 'NONE', *, *, #3894, .T. ) ;
#12832=EDGE_LOOP ( 'NONE', ( #5738, #5155, #7584, #10987 ) ) ;
#12833=ORIENTED_EDGE ( 'NONE', *, *, #1198, .F. ) ;
#12836=CARTESIAN_POINT ( 'NONE',  ( 175.9483885134608272, -179.3058001507315566, 84.88378295107887084 ) ) ;
#12838=VECTOR ( 'NONE', #3992, 1000.000000000000000 ) ;
#12839=EDGE_CURVE ( 'NONE', #3324, #13575, #9486, .T. ) ;
#12841=VECTOR ( 'NONE', #5783, 1000.000000000000114 ) ;
#12852=DIRECTION ( 'NONE',  ( 0.000000000000000000, 4.956352788505162775E-17, -1.000000000000000000 ) ) ;
#12853=CIRCLE ( 'NONE', #7903, 0.5000000000000004441 ) ;
#12867=ORIENTED_EDGE ( 'NONE', *, *, #2082, .F. ) ;
#12874=CARTESIAN_POINT ( 'NONE',  ( 190.0000000000000853, -178.6666270497714777, 53.18093594598651919 ) ) ;
#12875=EDGE_CURVE ( 'NONE', #5311, #13177, #11503, .T. ) ;
#12877=AXIS2_PLACEMENT_3D ( 'NONE', #6591, #15004, #15469 ) ;
#12884=EDGE_CURVE ( 'NONE', #8326, #8197, #12609, .T. ) ;
#12888=ORIENTED_EDGE ( 'NONE', *, *, #9833, .T. ) ;
#12892=EDGE_LOOP ( 'NONE', ( #14909, #6185, #6916, #632 ) ) ;
#12895=ORIENTED_EDGE ( 'NONE', *, *, #11169, .T. ) ;
#12904=ORIENTED_EDGE ( 'NONE', *, *, #5758, .F. ) ;
#12917=ORIENTED_EDGE ( 'NONE', *, *, #10394, .T. ) ;
#12918=CARTESIAN_POINT ( 'NONE',  ( 178.0000000000000853, -179.8058001507315566, 52.49999999999997868 ) ) ;
#12924=CARTESIAN_POINT ( 'NONE',  ( 175.9483885134608272, -179.3058001507315566, -29.88378295107906624 ) ) ;
#12935=SURFACE_STYLE_USAGE ( .BOTH. , #14348 ) ;
#12943=CARTESIAN_POINT ( 'NONE',  ( 177.5000000000000853, -178.7362136002515172, 52.68580191161573367 ) ) ;
#12948=DIRECTION ( 'NONE',  ( -0.000000000000000000, 1.000000000000000000, 0.000000000000000000 ) ) ;
#12955=DIRECTION ( 'NONE',  ( 0.000000000000000000, 0.000000000000000000, 1.000000000000000000 ) ) ;
#12958=CARTESIAN_POINT ( 'NONE',  ( -76.00000000000001421, -178.8058001507315566, -17.19066787724516843 ) ) ;
#12960=CARTESIAN_POINT ( 'NONE',  ( 178.0000000000000853, 15.03993994372673981, 10.05257423913146475 ) ) ;
#12962=DIRECTION ( 'NONE',  ( 0.000000000000000000, 0.000000000000000000, 1.000000000000000000 ) ) ;
#12964=EDGE_CURVE ( 'NONE', #15483, #7789, #4879, .T. ) ;
#12968=VERTEX_POINT ( 'NONE', #1944 ) ;
#12971=ORIENTED_EDGE ( 'NONE', *, *, #8548, .F. ) ;
#12972=CARTESIAN_POINT ( 'NONE',  ( -76.00000000000004263, 14.97035339324670744, 37.58005016923963382 ) ) ;
#12981=DIRECTION ( 'NONE',  ( 1.000000000000000000, 2.751328491981765035E-32, -3.965082230804130220E-16 ) ) ;
#12990=ORIENTED_EDGE ( 'NONE', *, *, #2736, .F. ) ;
#12991=DIRECTION ( 'NONE',  ( -0.000000000000000000, 1.000000000000000000, 6.938893903907227145E-17 ) ) ;
#12993=CARTESIAN_POINT ( 'NONE',  ( 184.0000000000000568, -181.3058001507315566, -41.45141194869120227 ) ) ;
#12998=DIRECTION ( 'NONE',  ( 0.000000000000000000, 0.000000000000000000, -1.000000000000000000 ) ) ;
#13001=CYLINDRICAL_SURFACE ( 'NONE', #2310, 0.4999999999999996114 ) ;
#13002=VERTEX_POINT ( 'NONE', #1229 ) ;
#13005=FACE_OUTER_BOUND ( 'NONE', #11274, .T. ) ;
#13009=CARTESIAN_POINT ( 'NONE',  ( 177.5000000000000853, -179.8058001507315566, 64.88378295107887084 ) ) ;
#13011=ORIENTED_EDGE ( 'NONE', *, *, #567, .F. ) ;
#13029=FACE_OUTER_BOUND ( 'NONE', #1106, .T. ) ;
#13031=LINE ( 'NONE', #7065, #5309 ) ;
#13032=CARTESIAN_POINT ( 'NONE',  ( 184.0000000000000568, 15.53993994372673626, 45.99999999999998579 ) ) ;
#13033=ORIENTED_EDGE ( 'NONE', *, *, #1479, .T. ) ;
#13039=CARTESIAN_POINT ( 'NONE',  ( -76.50000000000004263, 15.03993994372673804, 24.94742576086838781 ) ) ;
#13040=CARTESIAN_POINT ( 'NONE',  ( 190.0000000000000568, -179.8058001507315566, -17.19066787724516843 ) ) ;
#13041=EDGE_CURVE ( 'NONE', #10036, #12077, #4712, .T. ) ;
#13042=CIRCLE ( 'NONE', #8294, 0.5000000000000004441 ) ;
#13043=ORIENTED_EDGE ( 'NONE', *, *, #4535, .T. ) ;
#13050=CARTESIAN_POINT ( 'NONE',  ( -76.00000000000004263, -178.9449732516916072, 64.32815825124538378 ) ) ;
#13054=CIRCLE ( 'NONE', #5009, 1.000000000000000444 ) ;
#13060=EDGE_CURVE ( 'NONE', #1178, #12789, #11827, .T. ) ;
#13062=DIRECTION ( 'NONE',  ( 1.000000000000000000, -0.000000000000000000, -0.000000000000000000 ) ) ;
#13066=EDGE_CURVE ( 'NONE', #3832, #10070, #7661, .T. ) ;
#13076=DIRECTION ( 'NONE',  ( 0.000000000000000000, 0.9902680687415712502, 0.1391731009600584990 ) ) ;
#13083=DIRECTION ( 'NONE',  ( 0.000000000000000000, 1.000000000000000000, 6.938893903907227145E-17 ) ) ;
#13087=ORIENTED_EDGE ( 'NONE', *, *, #13202, .T. ) ;
#13088=CIRCLE ( 'NONE', #3029, 1.000000000000000888 ) ;
#13091=EDGE_CURVE ( 'NONE', #13177, #2407, #9877, .T. ) ;
#13098=ORIENTED_EDGE ( 'NONE', *, *, #14788, .F. ) ;
#13099=ORIENTED_EDGE ( 'NONE', *, *, #2285, .T. ) ;
#13101=DIRECTION ( 'NONE',  ( 5.518327896226369609E-17, 0.9902680687415712502, 0.1391731009600584990 ) ) ;
#13102=ADVANCED_FACE ( 'NONE', ( #11361 ), #12382, .F. ) ;
#13103=EDGE_LOOP ( 'NONE', ( #15554, #14915, #12463, #8308 ) ) ;
#13107=AXIS2_PLACEMENT_3D ( 'NONE', #2065, #1983, #3254 ) ;
#13108=AXIS2_PLACEMENT_3D ( 'NONE', #13142, #2344, #5976 ) ;
#13110=EDGE_LOOP ( 'NONE', ( #6572, #4116, #2444, #389 ) ) ;
#13111=DIRECTION ( 'NONE',  ( 1.000000000000000000, -0.000000000000000000, -0.000000000000000000 ) ) ;
#13112=CIRCLE ( 'NONE', #1265, 0.5000000000000004441 ) ;
#13114=CARTESIAN_POINT ( 'NONE',  ( 177.5000000000000853, 16.03993994372673981, 10.05257423913146475 ) ) ;
#13124=CYLINDRICAL_SURFACE ( 'NONE', #15509, 0.4999999999999996114 ) ;
#13125=DIRECTION ( 'NONE',  ( 0.000000000000000000, 1.734723475976805517E-15, 1.000000000000000000 ) ) ;
#13128=ORIENTED_EDGE ( 'NONE', *, *, #3338, .T. ) ;
#13133=CARTESIAN_POINT ( 'NONE',  ( -76.00000000000001421, -178.9449732516916072, -29.32815825124561471 ) ) ;
#13136=FACE_OUTER_BOUND ( 'NONE', #9793, .T. ) ;
#13138=AXIS2_PLACEMENT_3D ( 'NONE', #9342, #3333, #8171 ) ;
#13140=VERTEX_POINT ( 'NONE', #5600 ) ;
#13141=ORIENTED_EDGE ( 'NONE', *, *, #9952, .F. ) ;
#13142=CARTESIAN_POINT ( 'NONE',  ( 184.0000000000000568, -179.3058001507315566, -41.45141194869120227 ) ) ;
#13144=DIRECTION ( 'NONE',  ( 0.000000000000000000, -4.956352788505162775E-17, 1.000000000000000000 ) ) ;
#13145=DIRECTION ( 'NONE',  ( 1.000000000000000000, 0.000000000000000000, 0.000000000000000000 ) ) ;
#13150=EDGE_CURVE ( 'NONE', #4389, #9280, #1945, .T. ) ;
#13153=DIRECTION ( 'NONE',  ( 1.000000000000000000, 2.751328491981765035E-32, -3.965082230804130220E-16 ) ) ;
#13156=ADVANCED_FACE ( 'NONE', ( #12763 ), #7975, .T. ) ;
#13158=ORIENTED_EDGE ( 'NONE', *, *, #8099, .T. ) ;
#13160=DIRECTION ( 'NONE',  ( 0.000000000000000000, 0.1391731009600626345, 0.9902680687415706950 ) ) ;
#13171=DIRECTION ( 'NONE',  ( -1.000000000000000000, 0.000000000000000000, 0.000000000000000000 ) ) ;
#13172=ORIENTED_EDGE ( 'NONE', *, *, #6516, .T. ) ;
#13173=ADVANCED_FACE ( 'NONE', ( #13793, #8055 ), #3305, .T. ) ;
#13177=VERTEX_POINT ( 'NONE', #4320 ) ;
#13182=DIRECTION ( 'NONE',  ( -1.000000000000000000, 0.000000000000000000, 0.000000000000000000 ) ) ;
#13185=ORIENTED_EDGE ( 'NONE', *, *, #7671, .F. ) ;
#13189=FACE_OUTER_BOUND ( 'NONE', #1375, .T. ) ;
#13191=VERTEX_POINT ( 'NONE', #4238 ) ;
#13198=CARTESIAN_POINT ( 'NONE',  ( 175.9483885134608272, 15.53993994372673981, -2.500000000000070610 ) ) ;
#13202=EDGE_CURVE ( 'NONE', #3561, #4430, #1334, .T. ) ;
#13203=VERTEX_POINT ( 'NONE', #9078 ) ;
#13204=EDGE_CURVE ( 'NONE', #3026, #9812, #4472, .T. ) ;
#13210=DIRECTION ( 'NONE',  ( 0.000000000000000000, 1.000000000000000000, 6.938893903907227145E-17 ) ) ;
#13213=DIRECTION ( 'NONE',  ( 0.000000000000000000, 1.734723475976806306E-15, -1.000000000000000000 ) ) ;
#13214=ORIENTED_EDGE ( 'NONE', *, *, #4084, .F. ) ;
#13217=ORIENTED_EDGE ( 'NONE', *, *, #12205, .F. ) ;
#13218=ORIENTED_EDGE ( 'NONE', *, *, #6928, .T. ) ;
#13219=LINE ( 'NONE', #9611, #4282 ) ;
#13220=CARTESIAN_POINT ( 'NONE',  ( 177.5000000000000853, 15.53993994372673981, -17.50000000000002487 ) ) ;
#13222=FACE_OUTER_BOUND ( 'NONE', #11763, .T. ) ;
#13223=DIRECTION ( 'NONE',  ( 0.000000000000000000, 4.956352788505162775E-17, -1.000000000000000000 ) ) ;
#13224=CARTESIAN_POINT ( 'NONE',  ( -64.00000000000002842, 14.97035339324670744, 37.58005016923963382 ) ) ;
#13229=CIRCLE ( 'NONE', #361, 1.000000000000000000 ) ;
#13237=CARTESIAN_POINT ( 'NONE',  ( -76.00000000000001421, 16.03993994372673981, 24.94742576086838781 ) ) ;
#13242=EDGE_CURVE ( 'NONE', #234, #10853, #4620, .T. ) ;
#13253=ORIENTED_EDGE ( 'NONE', *, *, #6979, .T. ) ;
#13260=EDGE_CURVE ( 'NONE', #14171, #9678, #14439, .T. ) ;
#13262=EDGE_CURVE ( 'NONE', #4290, #10772, #6714, .T. ) ;
#13264=ORIENTED_EDGE ( 'NONE', *, *, #5883, .T. ) ;
#13267=ORIENTED_EDGE ( 'NONE', *, *, #10376, .F. ) ;
#13269=CARTESIAN_POINT ( 'NONE',  ( 184.0000000000000568, -201.3058001507315566, -41.45141194869120227 ) ) ;
#13272=ORIENTED_EDGE ( 'NONE', *, *, #2131, .F. ) ;
#13278=CARTESIAN_POINT ( 'NONE',  ( 178.0000000000000853, 13.40307322461931072, 37.29540324609171620 ) ) ;
#13284=DIRECTION ( 'NONE',  ( 1.000000000000000000, 0.000000000000000000, 0.000000000000000000 ) ) ;
#13285=DIRECTION ( 'NONE',  ( -5.518327896226364679E-17, -0.9902680687415713612, 0.1391731009600582492 ) ) ;
#13289=CARTESIAN_POINT ( 'NONE',  ( 178.0000000000000853, 14.90076684276668040, -2.084916134869000182 ) ) ;
#13290=ORIENTED_EDGE ( 'NONE', *, *, #4008, .F. ) ;
#13296=DIRECTION ( 'NONE',  ( -0.000000000000000000, -0.000000000000000000, 1.000000000000000000 ) ) ;
#13300=CARTESIAN_POINT ( 'NONE',  ( -63.50000000000002842, 14.90076684276667862, -2.084916134868993076 ) ) ;
#13303=VECTOR ( 'NONE', #9624, 1000.000000000000000 ) ;
#13305=FACE_OUTER_BOUND ( 'NONE', #14527, .T. ) ;
#13306=CARTESIAN_POINT ( 'NONE',  ( -76.50000000000001421, -181.3058001507315566, -51.45141194869120227 ) ) ;
#13307=LINE ( 'NONE', #10966, #1456 ) ;
#13315=DIRECTION ( 'NONE',  ( 0.000000000000000000, -1.000000000000000000, 0.000000000000000000 ) ) ;
#13317=DIRECTION ( 'NONE',  ( 0.000000000000000000, -1.734723475976808672E-15, -1.000000000000000000 ) ) ;
#13324=ORIENTED_EDGE ( 'NONE', *, *, #8264, .T. ) ;
#13326=ORIENTED_EDGE ( 'NONE', *, *, #14788, .T. ) ;
#13339=DIRECTION ( 'NONE',  ( 0.000000000000000000, 0.000000000000000000, 1.000000000000000000 ) ) ;
#13347=ORIENTED_EDGE ( 'NONE', *, *, #5273, .T. ) ;
#13348=EDGE_CURVE ( 'NONE', #7455, #4643, #13449, .T. ) ;
#13350=CARTESIAN_POINT ( 'NONE',  ( 178.0000000000000853, 16.03993994372673626, 52.49999999999997868 ) ) ;
#13353=ORIENTED_EDGE ( 'NONE', *, *, #7777, .F. ) ;
#13367=DIRECTION ( 'NONE',  ( 0.000000000000000000, -0.1391731009600592484, 0.9902680687415712502 ) ) ;
#13371=CARTESIAN_POINT ( 'NONE',  ( -76.50000000000004263, -179.8058001507315566, 84.88378295107887084 ) ) ;
#13386=DIRECTION ( 'NONE',  ( 1.000000000000000000, 0.000000000000000000, 0.000000000000000000 ) ) ;
#13388=CARTESIAN_POINT ( 'NONE',  ( -63.50000000000002842, 14.90076684276667862, 37.08491613486885541 ) ) ;
#13392=FACE_BOUND ( 'NONE', #2513, .T. ) ;
#13400=CARTESIAN_POINT ( 'NONE',  ( -76.00000000000004263, -178.7362136002515172, 52.68580191161573367 ) ) ;
#13402=DIRECTION ( 'NONE',  ( -1.000000000000000000, 0.000000000000000000, 0.000000000000000000 ) ) ;
#13409=EDGE_CURVE ( 'NONE', #8234, #5311, #10186, .T. ) ;
#13416=DIRECTION ( 'NONE',  ( -1.000000000000000000, 0.000000000000000000, 0.000000000000000000 ) ) ;
#13420=DIRECTION ( 'NONE',  ( 0.000000000000000000, 4.956352788505162775E-17, -1.000000000000000000 ) ) ;
#13426=VERTEX_POINT ( 'NONE', #6534 ) ;
#13427=DIRECTION ( 'NONE',  ( 0.000000000000000000, 0.000000000000000000, -1.000000000000000000 ) ) ;
#13433=ORIENTED_EDGE ( 'NONE', *, *, #10920, .F. ) ;
#13434=VERTEX_POINT ( 'NONE', #12510 ) ;
#13441=DIRECTION ( 'NONE',  ( 0.000000000000000000, 0.1391731009600592484, 0.9902680687415712502 ) ) ;
#13446=VERTEX_POINT ( 'NONE', #13388 ) ;
#13447=CARTESIAN_POINT ( 'NONE',  ( -63.50000000000002842, 15.53993994372673626, 52.49999999999997868 ) ) ;
#13449=CIRCLE ( 'NONE', #12692, 0.5000000000000004441 ) ;
#13452=VERTEX_POINT ( 'NONE', #2739 ) ;
#13455=VECTOR ( 'NONE', #5415, 1000.000000000000114 ) ;
#13460=CYLINDRICAL_SURFACE ( 'NONE', #7588, 1.500000000000001332 ) ;
#13461=AXIS2_PLACEMENT_3D ( 'NONE', #7188, #2504, #7339 ) ;
#13463=FACE_OUTER_BOUND ( 'NONE', #3017, .T. ) ;
#13464=ADVANCED_FACE ( 'NONE', ( #13463 ), #7723, .T. ) ;
#13468=LINE ( 'NONE', #2743, #7784 ) ;
#13469=FACE_BOUND ( 'NONE', #3882, .T. ) ;
#13471=FACE_OUTER_BOUND ( 'NONE', #1238, .T. ) ;
#13480=EDGE_LOOP ( 'NONE', ( #4113, #4407, #10926, #19 ) ) ;
#13482=CARTESIAN_POINT ( 'NONE',  ( -70.00000000000000000, 15.53993994372673981, -13.99999999999999112 ) ) ;
#13483=DIRECTION ( 'NONE',  ( 0.000000000000000000, -6.938893903907227145E-17, 1.000000000000000000 ) ) ;
#13485=ORIENTED_EDGE ( 'NONE', *, *, #310, .T. ) ;
#13490=CIRCLE ( 'NONE', #12736, 1.000000000000000888 ) ;
#13494=CARTESIAN_POINT ( 'NONE',  ( -76.00000000000001421, 15.53993994372673981, -17.50000000000002487 ) ) ;
#13496=CARTESIAN_POINT ( 'NONE',  ( 175.9483885134608272, 15.03993994372673981, -3.075184203610571654 ) ) ;
#13497=ORIENTED_EDGE ( 'NONE', *, *, #7017, .F. ) ;
#13499=ORIENTED_EDGE ( 'NONE', *, *, #2188, .T. ) ;
#13502=ORIENTED_EDGE ( 'NONE', *, *, #3354, .T. ) ;
#13503=DIRECTION ( 'NONE',  ( -1.000000000000000000, -0.000000000000000000, -0.000000000000000000 ) ) ;
#13507=VERTEX_POINT ( 'NONE', #9858 ) ;
#13508=CARTESIAN_POINT ( 'NONE',  ( 177.5000000000000853, 15.03993994372673981, -3.075184203610571654 ) ) ;
#13518=CARTESIAN_POINT ( 'NONE',  ( -64.00000000000002842, 21.51947656765318229, 9.953386152224130257 ) ) ;
#13524=FACE_OUTER_BOUND ( 'NONE', #260, .T. ) ;
#13529=ORIENTED_EDGE ( 'NONE', *, *, #6575, .T. ) ;
#13530=EDGE_CURVE ( 'NONE', #3126, #13507, #1626, .T. ) ;
#13540=ADVANCED_FACE ( 'NONE', ( #7563 ), #12362, .T. ) ;
#13541=CARTESIAN_POINT ( 'NONE',  ( 184.0000000000000568, 15.53993994372673981, -12.49999999999999289 ) ) ;
#13545=LINE ( 'NONE', #10022, #7024 ) ;
#13547=CARTESIAN_POINT ( 'NONE',  ( -63.50000000000002842, -179.8058001507315566, 64.88378295107887084 ) ) ;
#13550=EDGE_CURVE ( 'NONE', #10201, #4972, #11444, .T. ) ;
#13551=LINE ( 'NONE', #4813, #11100 ) ;
#13565=EDGE_CURVE ( 'NONE', #5473, #5101, #8819, .T. ) ;
#13567=CIRCLE ( 'NONE', #8043, 1.000000000000000888 ) ;
#13574=FACE_OUTER_BOUND ( 'NONE', #15090, .T. ) ;
#13575=VERTEX_POINT ( 'NONE', #12764 ) ;
#13577=ORIENTED_EDGE ( 'NONE', *, *, #8331, .F. ) ;
#13579=CARTESIAN_POINT ( 'NONE',  ( -76.00000000000001421, 15.03993994372673981, -2.075184203610571210 ) ) ;
#13587=DIRECTION ( 'NONE',  ( 1.000000000000000000, -0.000000000000000000, -0.000000000000000000 ) ) ;
#13589=EDGE_LOOP ( 'NONE', ( #2795, #3461, #5462, #14480 ) ) ;
#13591=CARTESIAN_POINT ( 'NONE',  ( -61.94838851346079167, -178.8058001507315566, -17.19066787724516843 ) ) ;
#13605=VERTEX_POINT ( 'NONE', #11281 ) ;
#13607=VECTOR ( 'NONE', #15086, 1000.000000000000000 ) ;
#13613=CARTESIAN_POINT ( 'NONE',  ( 178.0000000000000853, -178.8753867012115961, 64.82329228561619061 ) ) ;
#13616=ORIENTED_EDGE ( 'NONE', *, *, #15050, .F. ) ;
#13623=ADVANCED_FACE ( 'NONE', ( #12458 ), #4239, .T. ) ;
#13624=AXIS2_PLACEMENT_3D ( 'NONE', #9295, #7006, #12752 ) ;
#13626=ORIENTED_EDGE ( 'NONE', *, *, #6019, .T. ) ;
#13627=ORIENTED_EDGE ( 'NONE', *, *, #8664, .T. ) ;
#13628=CARTESIAN_POINT ( 'NONE',  ( -76.00000000000004263, -179.3058001507315566, 52.19066787724494816 ) ) ;
#13629=DIRECTION ( 'NONE',  ( 1.000000000000000000, 0.000000000000000000, 0.000000000000000000 ) ) ;
#13630=DIRECTION ( 'NONE',  ( 0.000000000000000000, 0.000000000000000000, -1.000000000000000000 ) ) ;
#13638=DIRECTION ( 'NONE',  ( 0.000000000000000000, 0.000000000000000000, 1.000000000000000000 ) ) ;
#13644=DIRECTION ( 'NONE',  ( -1.000000000000000000, -2.751328491981765035E-32, 3.965082230804130220E-16 ) ) ;
#13647=DIRECTION ( 'NONE',  ( 0.000000000000000000, 0.000000000000000000, -1.000000000000000000 ) ) ;
#13648=DIRECTION ( 'NONE',  ( 1.000000000000000000, 2.751328491981765035E-32, -3.965082230804130220E-16 ) ) ;
#13654=AXIS2_PLACEMENT_3D ( 'NONE', #582, #9212, #15029 ) ;
#13661=ORIENTED_EDGE ( 'NONE', *, *, #8534, .T. ) ;
#13664=DIRECTION ( 'NONE',  ( 0.000000000000000000, 4.956352788505162775E-17, -1.000000000000000000 ) ) ;
#13666=ORIENTED_EDGE ( 'NONE', *, *, #5758, .T. ) ;
#13667=LINE ( 'NONE', #14926, #11303 ) ;
#13678=DIRECTION ( 'NONE',  ( -3.965082230804130220E-16, 1.090924371466202084E-47, 1.000000000000000000 ) ) ;
#13679=EDGE_LOOP ( 'NONE', ( #4742, #10031, #5930, #3468 ) ) ;
#13688=ORIENTED_EDGE ( 'NONE', *, *, #6336, .T. ) ;
#13694=EDGE_CURVE ( 'NONE', #7467, #4995, #3077, .T. ) ;
#13705=CARTESIAN_POINT ( 'NONE',  ( -64.00000000000002842, 16.03993994372673981, 10.05257423913146475 ) ) ;
#13706=VECTOR ( 'NONE', #10482, 1000.000000000000000 ) ;
#13710=CARTESIAN_POINT ( 'NONE',  ( -61.94838851346079167, 15.03993994372673981, -3.075184203610571654 ) ) ;
#13714=CARTESIAN_POINT ( 'NONE',  ( -76.00000000000004263, 15.53993994372673804, 52.49999999999997868 ) ) ;
#13721=CARTESIAN_POINT ( 'NONE',  ( 190.5000000000000568, -178.8058001507315566, -30.31842631998718574 ) ) ;
#13723=ORIENTED_EDGE ( 'NONE', *, *, #14218, .T. ) ;
#13726=ORIENTED_EDGE ( 'NONE', *, *, #6558, .F. ) ;
#13729=ORIENTED_EDGE ( 'NONE', *, *, #11900, .F. ) ;
#13732=VECTOR ( 'NONE', #8255, 1000.000000000000000 ) ;
#13734=PLANE ( 'NONE',  #13931 ) ;
#13743=ORIENTED_EDGE ( 'NONE', *, *, #9302, .F. ) ;
#13745=ADVANCED_FACE ( 'NONE', ( #7976 ), #6915, .T. ) ;
#13750=CARTESIAN_POINT ( 'NONE',  ( -70.00000000000000000, -179.3058001507315566, -41.45141194869120227 ) ) ;
#13751=LINE ( 'NONE', #797, #12751 ) ;
#13754=EDGE_CURVE ( 'NONE', #12671, #11360, #4989, .T. ) ;
#13756=CIRCLE ( 'NONE', #14261, 1.000000000000000888 ) ;
#13761=CARTESIAN_POINT ( 'NONE',  ( 175.9483885134608272, -179.3058001507315566, -51.45141194869120227 ) ) ;
#13762=LINE ( 'NONE', #12569, #4923 ) ;
#13768=ORIENTED_EDGE ( 'NONE', *, *, #2167, .T. ) ;
#13770=AXIS2_PLACEMENT_3D ( 'NONE', #7480, #1380, #14559 ) ;
#13771=EDGE_CURVE ( 'NONE', #6271, #6990, #9536, .T. ) ;
#13775=DIRECTION ( 'NONE',  ( 0.000000000000000000, 0.000000000000000000, 1.000000000000000000 ) ) ;
#13777=EDGE_LOOP ( 'NONE', ( #15334, #5394, #6681, #14015 ) ) ;
#13778=FACE_OUTER_BOUND ( 'NONE', #2328, .T. ) ;
#13788=DIRECTION ( 'NONE',  ( -0.000000000000000000, 6.938893903907227145E-17, -1.000000000000000000 ) ) ;
#13793=FACE_BOUND ( 'NONE', #69, .T. ) ;
#13796=DIRECTION ( 'NONE',  ( 0.000000000000000000, -1.000000000000000000, 0.000000000000000000 ) ) ;
#13797=VERTEX_POINT ( 'NONE', #5983 ) ;
#13801=ORIENTED_EDGE ( 'NONE', *, *, #12594, .T. ) ;
#13803=CARTESIAN_POINT ( 'NONE',  ( 184.0000000000000568, -201.3058001507315566, -39.95141194869120937 ) ) ;
#13804=ORIENTED_EDGE ( 'NONE', *, *, #8221, .T. ) ;
#13809=AXIS2_PLACEMENT_3D ( 'NONE', #9260, #12948, #14284 ) ;
#13827=AXIS2_PLACEMENT_3D ( 'NONE', #13289, #11179, #331 ) ;
#13832=CARTESIAN_POINT ( 'NONE',  ( 190.0000000000000853, 15.53993994372673804, 38.07518420361041933 ) ) ;
#13834=CIRCLE ( 'NONE', #4766, 0.5000000000000004441 ) ;
#13837=AXIS2_PLACEMENT_3D ( 'NONE', #6349, #1746, #4115 ) ;
#13844=ORIENTED_EDGE ( 'NONE', *, *, #5883, .F. ) ;
#13848=CIRCLE ( 'NONE', #7057, 1.000000000000000000 ) ;
#13850=EDGE_CURVE ( 'NONE', #4671, #2454, #11948, .T. ) ;
#13851=AXIS2_PLACEMENT_3D ( 'NONE', #14206, #15464, #1975 ) ;
#13853=CYLINDRICAL_SURFACE ( 'NONE', #12492, 0.5000000000000004441 ) ;
#13854=DIRECTION ( 'NONE',  ( 3.965082230804130220E-16, 1.090924371466202084E-47, 1.000000000000000000 ) ) ;
#13855=CIRCLE ( 'NONE', #7067, 0.5000000000000004441 ) ;
#13858=FACE_OUTER_BOUND ( 'NONE', #1814, .T. ) ;
#13859=VERTEX_POINT ( 'NONE', #3726 ) ;
#13864=ADVANCED_FACE ( 'NONE', ( #2461 ), #14061, .T. ) ;
#13870=VERTEX_POINT ( 'NONE', #2549 ) ;
#13871=VERTEX_POINT ( 'NONE', #2628 ) ;
#13873=CARTESIAN_POINT ( 'NONE',  ( -63.50000000000002842, -179.3753867012115961, -29.38864891670827362 ) ) ;
#13874=DIRECTION ( 'NONE',  ( -0.000000000000000000, 1.000000000000000000, 0.000000000000000000 ) ) ;
#13875=TOROIDAL_SURFACE ( 'NONE', #3788, 1.000000000000000000, 0.5000000000000000000 ) ;
#13880=EDGE_CURVE ( 'NONE', #12081, #13177, #7761, .T. ) ;
#13881=CARTESIAN_POINT ( 'NONE',  ( -76.00000000000001421, -179.8058001507315566, -17.50000000000002487 ) ) ;
#13884=LINE ( 'NONE', #2194, #7586 ) ;
#13892=DIRECTION ( 'NONE',  ( -1.000000000000000000, 0.000000000000000000, -0.000000000000000000 ) ) ;
#13893=CARTESIAN_POINT ( 'NONE',  ( -64.00000000000002842, 15.03993994372673981, -3.075184203610571654 ) ) ;
#13898=ORIENTED_EDGE ( 'NONE', *, *, #1764, .F. ) ;
#13905=VECTOR ( 'NONE', #14423, 1000.000000000000000 ) ;
#13908=ORIENTED_EDGE ( 'NONE', *, *, #2798, .F. ) ;
#13911=CARTESIAN_POINT ( 'NONE',  ( 178.0000000000000853, -179.3058001507315566, -30.31842631998718574 ) ) ;
#13917=CYLINDRICAL_SURFACE ( 'NONE', #5957, 0.5000000000000004441 ) ;
#13921=CARTESIAN_POINT ( 'NONE',  ( -76.50000000000001421, 16.03993994372673981, 10.05257423913146475 ) ) ;
#13924=PLANE ( 'NONE',  #5429 ) ;
#13926=CARTESIAN_POINT ( 'NONE',  ( -76.00000000000001421, -178.8058001507315566, -17.19066787724516843 ) ) ;
#13931=AXIS2_PLACEMENT_3D ( 'NONE', #5143, #2937, #11224 ) ;
#13933=DIRECTION ( 'NONE',  ( 0.000000000000000000, -0.1391731009600592484, 0.9902680687415712502 ) ) ;
#13935=CARTESIAN_POINT ( 'NONE',  ( 178.0000000000000853, 15.17911304468679745, 25.93769382960995529 ) ) ;
#13939=ORIENTED_EDGE ( 'NONE', *, *, #3168, .F. ) ;
#13956=EDGE_CURVE ( 'NONE', #10772, #4850, #3720, .T. ) ;
#13957=EDGE_CURVE ( 'NONE', #13797, #11925, #12533, .T. ) ;
#13958=EDGE_CURVE ( 'NONE', #8697, #8310, #7015, .T. ) ;
#13963=FACE_OUTER_BOUND ( 'NONE', #2510, .T. ) ;
#13967=ORIENTED_EDGE ( 'NONE', *, *, #4482, .F. ) ;
#13969=CYLINDRICAL_SURFACE ( 'NONE', #9886, 0.5000000000000004441 ) ;
#13972=CARTESIAN_POINT ( 'NONE',  ( 190.0000000000000568, 16.03993994372673981, -7.458121719691109004E-14 ) ) ;
#13974=DIRECTION ( 'NONE',  ( 0.000000000000000000, 0.000000000000000000, 1.000000000000000000 ) ) ;
#13978=ORIENTED_EDGE ( 'NONE', *, *, #10517, .F. ) ;
#13995=ORIENTED_EDGE ( 'NONE', *, *, #15050, .T. ) ;
#14004=AXIS2_PLACEMENT_3D ( 'NONE', #10356, #15151, #10277 ) ;
#14005=LINE ( 'NONE', #8025, #6412 ) ;
#14006=DIRECTION ( 'NONE',  ( -3.965082230804130220E-16, 1.090924371466202084E-47, 1.000000000000000000 ) ) ;
#14007=FACE_OUTER_BOUND ( 'NONE', #14545, .T. ) ;
#14008=VERTEX_POINT ( 'NONE', #3887 ) ;
#14011=DIRECTION ( 'NONE',  ( -0.000000000000000000, 0.9902680687415712502, 0.1391731009600584990 ) ) ;
#14013=DIRECTION ( 'NONE',  ( 0.000000000000000000, 0.000000000000000000, -1.000000000000000000 ) ) ;
#14014=FACE_OUTER_BOUND ( 'NONE', #12892, .T. ) ;
#14015=ORIENTED_EDGE ( 'NONE', *, *, #10533, .F. ) ;
#14022=DIRECTION ( 'NONE',  ( 1.000000000000000000, 0.000000000000000000, 0.000000000000000000 ) ) ;
#14024=PLANE ( 'NONE',  #6242 ) ;
#14029=CARTESIAN_POINT ( 'NONE',  ( 190.0000000000000568, -178.8058001507315566, -17.19066787724516843 ) ) ;
#14031=CARTESIAN_POINT ( 'NONE',  ( 177.5000000000000853, -178.8058001507315566, -17.19066787724516843 ) ) ;
#14034=ORIENTED_EDGE ( 'NONE', *, *, #6558, .T. ) ;
#14041=CYLINDRICAL_SURFACE ( 'NONE', #5815, 0.5000000000000004441 ) ;
#14042=EDGE_CURVE ( 'NONE', #13140, #5266, #9782, .T. ) ;
#14043=DIRECTION ( 'NONE',  ( -0.000000000000000000, 0.9902680687415702510, 0.1391731009600660485 ) ) ;
#14048=VERTEX_POINT ( 'NONE', #3384 ) ;
#14059=DIRECTION ( 'NONE',  ( 0.000000000000000000, 0.000000000000000000, -1.000000000000000000 ) ) ;
#14061=TOROIDAL_SURFACE ( 'NONE', #2471, 1.000000000000000000, 0.5000000000000000000 ) ;
#14062=DIRECTION ( 'NONE',  ( 0.000000000000000000, 1.000000000000000000, 6.938893903907227145E-17 ) ) ;
#14063=DIRECTION ( 'NONE',  ( -0.000000000000000000, 1.000000000000000000, 6.938893903907227145E-17 ) ) ;
#14064=LINE ( 'NONE', #877, #478 ) ;
#14067=DIRECTION ( 'NONE',  ( -1.000000000000000000, 0.000000000000000000, 0.000000000000000000 ) ) ;
#14070=FACE_BOUND ( 'NONE', #7508, .T. ) ;
#14074=ORIENTED_EDGE ( 'NONE', *, *, #12208, .F. ) ;
#14077=ORIENTED_EDGE ( 'NONE', *, *, #14081, .F. ) ;
#14078=DIRECTION ( 'NONE',  ( 1.000000000000000000, 0.000000000000000000, 0.000000000000000000 ) ) ;
#14081=EDGE_CURVE ( 'NONE', #9280, #4290, #10042, .T. ) ;
#14084=DIRECTION ( 'NONE',  ( 5.518327896226369609E-17, -0.9902680687415712502, -0.1391731009600584990 ) ) ;
#14086=DIRECTION ( 'NONE',  ( -0.000000000000000000, 1.000000000000000000, -0.000000000000000000 ) ) ;
#14088=AXIS2_PLACEMENT_3D ( 'NONE', #13750, #2799, #11241 ) ;
#14089=DIRECTION ( 'NONE',  ( 3.965082230804130220E-16, -4.956352788505162775E-17, 1.000000000000000000 ) ) ;
#14096=DIRECTION ( 'NONE',  ( 0.000000000000000000, 0.000000000000000000, 1.000000000000000000 ) ) ;
#14098=FACE_OUTER_BOUND ( 'NONE', #2226, .T. ) ;
#14102=CARTESIAN_POINT ( 'NONE',  ( -70.00000000000000000, -179.3058001507315566, -41.45141194869120227 ) ) ;
#14103=CARTESIAN_POINT ( 'NONE',  ( 178.0000000000000853, -178.8058001507315566, -30.31842631998718574 ) ) ;
#14105=ADVANCED_FACE ( 'NONE', ( #9388 ), #2209, .T. ) ;
#14108=VECTOR ( 'NONE', #2538, 1000.000000000000000 ) ;
#14109=CARTESIAN_POINT ( 'NONE',  ( -64.00000000000002842, 15.53993994372673981, -2.500000000000070610 ) ) ;
#14110=ORIENTED_EDGE ( 'NONE', *, *, #8947, .T. ) ;
#14116=CARTESIAN_POINT ( 'NONE',  ( -76.00000000000001421, 15.03993994372673981, -3.075184203610571654 ) ) ;
#14118=ORIENTED_EDGE ( 'NONE', *, *, #8412, .T. ) ;
#14120=DIRECTION ( 'NONE',  ( 1.000000000000000000, 0.000000000000000000, 3.965082230804112963E-16 ) ) ;
#14124=VECTOR ( 'NONE', #5714, 1000.000000000000000 ) ;
#14125=ADVANCED_FACE ( 'NONE', ( #7190 ), #2272, .T. ) ;
#14126=VECTOR ( 'NONE', #4375, 1000.000000000000000 ) ;
#14127=EDGE_LOOP ( 'NONE', ( #13801, #118, #12485, #5920 ) ) ;
#14128=DIRECTION ( 'NONE',  ( 0.000000000000000000, 0.000000000000000000, -1.000000000000000000 ) ) ;
#14129=EDGE_LOOP ( 'NONE', ( #5076, #5838, #11897, #11448 ) ) ;
#14131=DIRECTION ( 'NONE',  ( 0.000000000000000000, 4.956352788505162775E-17, -1.000000000000000000 ) ) ;
#14132=CARTESIAN_POINT ( 'NONE',  ( 178.0000000000000853, 15.03993994372673981, 10.05257423913146475 ) ) ;
#14136=DIRECTION ( 'NONE',  ( -0.000000000000000000, -0.9902680687415710281, 0.1391731009600611635 ) ) ;
#14138=AXIS2_PLACEMENT_3D ( 'NONE', #3292, #15344, #3206 ) ;
#14140=DIRECTION ( 'NONE',  ( -1.000000000000000000, 0.000000000000000000, 3.965082230804112963E-16 ) ) ;
#14146=VECTOR ( 'NONE', #4020, 1000.000000000000000 ) ;
#14158=CYLINDRICAL_SURFACE ( 'NONE', #9320, 0.5000000000000004441 ) ;
#14166=DIRECTION ( 'NONE',  ( 1.000000000000000000, 0.000000000000000000, -0.000000000000000000 ) ) ;
#14170=CARTESIAN_POINT ( 'NONE',  ( 184.0000000000000568, -179.3058001507315566, -39.95141194869120937 ) ) ;
#14171=VERTEX_POINT ( 'NONE', #7104 ) ;
#14172=EDGE_LOOP ( 'NONE', ( #14538, #4781, #2245, #11602, #11273, #2546, #14303, #6652, #10261 ) ) ;
#14182=CARTESIAN_POINT ( 'NONE',  ( 190.0000000000000568, -178.9449732516916072, -29.32815825124561471 ) ) ;
#14190=EDGE_CURVE ( 'NONE', #4326, #13434, #14340, .T. ) ;
#14191=CARTESIAN_POINT ( 'NONE',  ( 177.5000000000000853, 15.53993994372673981, -3.075184203610571654 ) ) ;
#14198=ADVANCED_FACE ( 'NONE', ( #5751, #7262 ), #12707, .T. ) ;
#14199=VERTEX_POINT ( 'NONE', #10569 ) ;
#14206=CARTESIAN_POINT ( 'NONE',  ( -76.00000000000004263, 16.03993994372673626, 38.07518420361041933 ) ) ;
#14212=EDGE_CURVE ( 'NONE', #7455, #2394, #8792, .T. ) ;
#14213=ORIENTED_EDGE ( 'NONE', *, *, #15381, .F. ) ;
#14215=VECTOR ( 'NONE', #8220, 1000.000000000000000 ) ;
#14218=EDGE_CURVE ( 'NONE', #6739, #10201, #1550, .T. ) ;
#14220=LINE ( 'NONE', #3417, #6564 ) ;
#14223=DIRECTION ( 'NONE',  ( 0.000000000000000000, 1.000000000000000000, 6.938893903907227145E-17 ) ) ;
#14227=ORIENTED_EDGE ( 'NONE', *, *, #3577, .T. ) ;
#14230=ORIENTED_EDGE ( 'NONE', *, *, #310, .F. ) ;
#14232=EDGE_CURVE ( 'NONE', #831, #592, #13468, .T. ) ;
#14233=EDGE_CURVE ( 'NONE', #7696, #10895, #7419, .T. ) ;
#14234=CARTESIAN_POINT ( 'NONE',  ( 190.0000000000000568, 16.03993994372673981, -7.458121719691109004E-14 ) ) ;
#14242=ORIENTED_EDGE ( 'NONE', *, *, #9891, .T. ) ;
#14245=CARTESIAN_POINT ( 'NONE',  ( -76.00000000000001421, 15.53993994372673804, 25.38206912977649310 ) ) ;
#14246=DIRECTION ( 'NONE',  ( 0.000000000000000000, 0.000000000000000000, 1.000000000000000000 ) ) ;
#14261=AXIS2_PLACEMENT_3D ( 'NONE', #1798, #14968, #10408 ) ;
#14263=CYLINDRICAL_SURFACE ( 'NONE', #9706, 0.5000000000000004441 ) ;
#14265=DIRECTION ( 'NONE',  ( 0.000000000000000000, 0.000000000000000000, -1.000000000000000000 ) ) ;
#14268=ORIENTED_EDGE ( 'NONE', *, *, #3965, .F. ) ;
#14275=ORIENTED_EDGE ( 'NONE', *, *, #12268, .F. ) ;
#14278=ADVANCED_FACE ( 'NONE', ( #6224 ), #182, .T. ) ;
#14282=DIRECTION ( 'NONE',  ( 0.000000000000000000, 0.000000000000000000, -1.000000000000000000 ) ) ;
#14284=DIRECTION ( 'NONE',  ( 0.000000000000000000, -0.000000000000000000, 1.000000000000000000 ) ) ;
#14285=EDGE_LOOP ( 'NONE', ( #3694, #12904, #2078, #6588 ) ) ;
#14291=CARTESIAN_POINT ( 'NONE',  ( 175.9483885134608272, -181.3058001507315566, 84.88378295107885663 ) ) ;
#14295=EDGE_CURVE ( 'NONE', #2689, #12599, #13307, .T. ) ;
#14296=LINE ( 'NONE', #2229, #108 ) ;
#14303=ORIENTED_EDGE ( 'NONE', *, *, #13694, .T. ) ;
#14304=DIRECTION ( 'NONE',  ( 0.000000000000000000, 1.000000000000000000, 6.938893903907227145E-17 ) ) ;
#14315=ORIENTED_EDGE ( 'NONE', *, *, #15205, .T. ) ;
#14319=FACE_OUTER_BOUND ( 'NONE', #12296, .T. ) ;
#14321=AXIS2_PLACEMENT_3D ( 'NONE', #12874, #4351, #10361 ) ;
#14324=CARTESIAN_POINT ( 'NONE',  ( 190.0000000000000853, 15.53993994372673626, 52.49999999999997868 ) ) ;
#14327=CIRCLE ( 'NONE', #7040, 0.5000000000000004441 ) ;
#14328=LINE ( 'NONE', #2422, #5402 ) ;
#14333=ADVANCED_FACE ( 'NONE', ( #8595, #13392 ), #12211, .F. ) ;
#14338=DIRECTION ( 'NONE',  ( -0.000000000000000000, 1.000000000000000000, 6.938893903907227145E-17 ) ) ;
#14340=LINE ( 'NONE', #5830, #13303 ) ;
#14342=ORIENTED_EDGE ( 'NONE', *, *, #14232, .F. ) ;
#14344=FACE_OUTER_BOUND ( 'NONE', #9354, .T. ) ;
#14346=( GEOMETRIC_REPRESENTATION_CONTEXT ( 3 ) GLOBAL_UNCERTAINTY_ASSIGNED_CONTEXT ( ( #6913 ) ) GLOBAL_UNIT_ASSIGNED_CONTEXT ( ( #248, #12111, #14632 ) ) REPRESENTATION_CONTEXT ( 'NONE', 'WORKASPACE' ) );
#14347=DIRECTION ( 'NONE',  ( 1.000000000000000000, 2.751328491981765035E-32, -3.965082230804130220E-16 ) ) ;
#14348=SURFACE_SIDE_STYLE ('',( #9548 ) ) ;
#14350=DIRECTION ( 'NONE',  ( 0.000000000000000000, 0.000000000000000000, -1.000000000000000000 ) ) ;
#14351=DIRECTION ( 'NONE',  ( 0.000000000000000000, 0.000000000000000000, 1.000000000000000000 ) ) ;
#14352=ADVANCED_FACE ( 'NONE', ( #12593 ), #11505, .T. ) ;
#14353=ORIENTED_EDGE ( 'NONE', *, *, #3168, .T. ) ;
#14354=TOROIDAL_SURFACE ( 'NONE', #9836, 1.000000000000000000, 0.5000000000000000000 ) ;
#14360=VERTEX_POINT ( 'NONE', #1704 ) ;
#14366=CARTESIAN_POINT ( 'NONE',  ( 190.0000000000000568, -179.3058001507315566, -51.45141194869120937 ) ) ;
#14371=CIRCLE ( 'NONE', #13108, 1.499999999999994449 ) ;
#14372=EDGE_CURVE ( 'NONE', #3478, #12658, #10054, .T. ) ;
#14375=ORIENTED_EDGE ( 'NONE', *, *, #11680, .T. ) ;
#14376=AXIS2_PLACEMENT_3D ( 'NONE', #6881, #9322, #689 ) ;
#14377=ORIENTED_EDGE ( 'NONE', *, *, #14690, .T. ) ;
#14380=DIRECTION ( 'NONE',  ( 0.000000000000000000, -1.000000000000000000, -4.956352788505160310E-17 ) ) ;
#14381=DIRECTION ( 'NONE',  ( 0.000000000000000000, 0.000000000000000000, 1.000000000000000000 ) ) ;
#14383=ORIENTED_EDGE ( 'NONE', *, *, #7254, .T. ) ;
#14388=DIRECTION ( 'NONE',  ( 0.000000000000000000, -0.1391731009600592484, -0.9902680687415712502 ) ) ;
#14390=AXIS2_PLACEMENT_3D ( 'NONE', #10212, #5475, #11629 ) ;
#14401=VERTEX_POINT ( 'NONE', #7728 ) ;
#14407=AXIS2_PLACEMENT_3D ( 'NONE', #1101, #4580, #15531 ) ;
#14409=CARTESIAN_POINT ( 'NONE',  ( 190.5000000000000853, -178.8058001507315566, 52.19066787724494816 ) ) ;
#14411=CARTESIAN_POINT ( 'NONE',  ( 178.0000000000000853, 16.03993994372673981, 7.553451883674125344E-16 ) ) ;
#14413=LINE ( 'NONE', #2660, #7337 ) ;
#14417=DIRECTION ( 'NONE',  ( 1.000000000000000000, -2.751328491981765035E-32, 3.965082230804130220E-16 ) ) ;
#14418=DIRECTION ( 'NONE',  ( -1.000000000000000000, 0.000000000000000000, 0.000000000000000000 ) ) ;
#14423=DIRECTION ( 'NONE',  ( 1.000000000000000000, 0.000000000000000000, 0.000000000000000000 ) ) ;
#14424=CARTESIAN_POINT ( 'NONE',  ( -70.00000000000000000, -181.3058001507315566, -42.95141194869119516 ) ) ;
#14427=DIRECTION ( 'NONE',  ( 0.000000000000000000, 0.000000000000000000, -1.000000000000000000 ) ) ;
#14428=EDGE_CURVE ( 'NONE', #9410, #14199, #15066, .T. ) ;
#14429=EDGE_CURVE ( 'NONE', #11107, #3604, #6270, .T. ) ;
#14432=CARTESIAN_POINT ( 'NONE',  ( -64.00000000000002842, 15.53993994372673981, -17.50000000000002487 ) ) ;
#14434=VERTEX_POINT ( 'NONE', #10164 ) ;
#14435=ORIENTED_EDGE ( 'NONE', *, *, #4399, .F. ) ;
#14438=ORIENTED_EDGE ( 'NONE', *, *, #8534, .F. ) ;
#14439=CIRCLE ( 'NONE', #6407, 0.5000000000000004441 ) ;
#14441=ORIENTED_EDGE ( 'NONE', *, *, #1489, .F. ) ;
#14442=VERTEX_POINT ( 'NONE', #10086 ) ;
#14446=PLANE ( 'NONE',  #4645 ) ;
#14451=CIRCLE ( 'NONE', #4898, 1.000000000000000888 ) ;
#14452=CYLINDRICAL_SURFACE ( 'NONE', #1112, 1.499999999999994449 ) ;
#14455=DIRECTION ( 'NONE',  ( 0.000000000000000000, 0.000000000000000000, -1.000000000000000000 ) ) ;
#14456=ADVANCED_FACE ( 'NONE', ( #11269 ), #4074, .F. ) ;
#14463=ORIENTED_EDGE ( 'NONE', *, *, #13041, .F. ) ;
#14465=DIRECTION ( 'NONE',  ( -1.000000000000000000, 0.000000000000000000, 0.000000000000000000 ) ) ;
#14466=CARTESIAN_POINT ( 'NONE',  ( -76.00000000000004263, 21.51947656765315386, 25.04661384777570987 ) ) ;
#14474=LINE ( 'NONE', #3438, #14985 ) ;
#14477=ORIENTED_EDGE ( 'NONE', *, *, #7764, .T. ) ;
#14480=ORIENTED_EDGE ( 'NONE', *, *, #11926, .F. ) ;
#14482=CARTESIAN_POINT ( 'NONE',  ( -63.50000000000002842, 15.53993994372673804, 24.94742576086838781 ) ) ;
#14486=FACE_OUTER_BOUND ( 'NONE', #3371, .T. ) ;
#14487=CARTESIAN_POINT ( 'NONE',  ( 190.0000000000000853, 14.97035339324670744, 37.58005016923963382 ) ) ;
#14490=CARTESIAN_POINT ( 'NONE',  ( -64.00000000000002842, 15.53993994372673981, 25.38206912977650376 ) ) ;
#14495=DIRECTION ( 'NONE',  ( 0.000000000000000000, 0.000000000000000000, -1.000000000000000000 ) ) ;
#14496=ORIENTED_EDGE ( 'NONE', *, *, #5152, .T. ) ;
#14499=CARTESIAN_POINT ( 'NONE',  ( -76.50000000000001421, -178.6666270497714777, -18.18093594598673945 ) ) ;
#14508=VECTOR ( 'NONE', #2970, 1000.000000000000114 ) ;
#14509=EDGE_CURVE ( 'NONE', #7288, #8073, #3735, .T. ) ;
#14517=ORIENTED_EDGE ( 'NONE', *, *, #7183, .T. ) ;
#14522=EDGE_LOOP ( 'NONE', ( #12990, #7910, #12621, #8063 ) ) ;
#14523=CARTESIAN_POINT ( 'NONE',  ( -76.50000000000001421, -179.3058001507315566, -30.31842631998718574 ) ) ;
#14524=DIRECTION ( 'NONE',  ( 0.000000000000000000, 0.1391731009600592484, 0.9902680687415712502 ) ) ;
#14527=EDGE_LOOP ( 'NONE', ( #4566, #9746, #4411, #945 ) ) ;
#14529=EDGE_CURVE ( 'NONE', #15193, #2866, #11309, .T. ) ;
#14538=ORIENTED_EDGE ( 'NONE', *, *, #1181, .F. ) ;
#14539=CARTESIAN_POINT ( 'NONE',  ( -61.94838851346079167, -178.8058001507315566, -30.31842631998718574 ) ) ;
#14542=EDGE_CURVE ( 'NONE', #3604, #8586, #10476, .T. ) ;
#14545=EDGE_LOOP ( 'NONE', ( #10543, #12388, #5288, #7749, #13267, #11848, #1120, #10402, #7593, #13804, #15454, #5391, #15376, #11102, #1353, #7510, #11660 ) ) ;
#14550=CARTESIAN_POINT ( 'NONE',  ( -70.00000000000000000, 15.53993994372673626, 47.49999999999997868 ) ) ;
#14555=LINE ( 'NONE', #10713, #9346 ) ;
#14556=CARTESIAN_POINT ( 'NONE',  ( -76.00000000000007105, -178.8058001507315566, 65.31842631998698323 ) ) ;
#14558=DIRECTION ( 'NONE',  ( 0.000000000000000000, 1.000000000000000000, 0.000000000000000000 ) ) ;
#14559=DIRECTION ( 'NONE',  ( -3.965082230804130220E-16, 1.090924371466202084E-47, 1.000000000000000000 ) ) ;
#14562=AXIS2_PLACEMENT_3D ( 'NONE', #10650, #7648, #7341 ) ;
#14568=CIRCLE ( 'NONE', #2227, 0.5000000000000004441 ) ;
#14571=ORIENTED_EDGE ( 'NONE', *, *, #4767, .F. ) ;
#14575=ORIENTED_EDGE ( 'NONE', *, *, #11033, .F. ) ;
#14579=CARTESIAN_POINT ( 'NONE',  ( -64.00000000000002842, 16.03993994372673981, 7.553451883674125344E-16 ) ) ;
#14583=VECTOR ( 'NONE', #1711, 1000.000000000000000 ) ;
#14585=VERTEX_POINT ( 'NONE', #6852 ) ;
#14586=CIRCLE ( 'NONE', #12326, 0.5000000000000004441 ) ;
#14591=ORIENTED_EDGE ( 'NONE', *, *, #6450, .T. ) ;
#14596=LINE ( 'NONE', #3796, #11829 ) ;
#14604=CARTESIAN_POINT ( 'NONE',  ( 190.5000000000000568, -178.6666270497714777, -18.18093594598673945 ) ) ;
#14606=CIRCLE ( 'NONE', #7562, 0.5000000000000004441 ) ;
#14617=ORIENTED_EDGE ( 'NONE', *, *, #11908, .F. ) ;
#14621=ORIENTED_EDGE ( 'NONE', *, *, #12884, .F. ) ;
#14624=LINE ( 'NONE', #241, #8980 ) ;
#14628=DIRECTION ( 'NONE',  ( 1.000000000000000000, -0.000000000000000000, -0.000000000000000000 ) ) ;
#14630=ORIENTED_EDGE ( 'NONE', *, *, #12610, .F. ) ;
#14631=AXIS2_PLACEMENT_3D ( 'NONE', #8990, #8827, #3857 ) ;
#14632=( NAMED_UNIT ( * ) SI_UNIT ( $, .STERADIAN. ) SOLID_ANGLE_UNIT ( ) );
#14634=ORIENTED_EDGE ( 'NONE', *, *, #10517, .T. ) ;
#14635=PLANE ( 'NONE',  #4576 ) ;
#14638=CYLINDRICAL_SURFACE ( 'NONE', #8802, 0.4999999999999996114 ) ;
#14642=ORIENTED_EDGE ( 'NONE', *, *, #2285, .F. ) ;
#14644=CIRCLE ( 'NONE', #14138, 0.5000000000000004441 ) ;
#14645=DIRECTION ( 'NONE',  ( -1.000000000000000000, 0.000000000000000000, 0.000000000000000000 ) ) ;
#14659=EDGE_LOOP ( 'NONE', ( #5894, #14118 ) ) ;
#14660=DIRECTION ( 'NONE',  ( 0.000000000000000000, 0.000000000000000000, 1.000000000000000000 ) ) ;
#14662=DIRECTION ( 'NONE',  ( 0.000000000000000000, 1.000000000000000000, 0.000000000000000000 ) ) ;
#14664=CIRCLE ( 'NONE', #8139, 0.5000000000000004441 ) ;
#14668=VERTEX_POINT ( 'NONE', #10787 ) ;
#14675=CIRCLE ( 'NONE', #561, 0.5000000000000004441 ) ;
#14681=EDGE_CURVE ( 'NONE', #13871, #6214, #10546, .T. ) ;
#14682=LINE ( 'NONE', #14986, #3097 ) ;
#14687=ORIENTED_EDGE ( 'NONE', *, *, #3081, .T. ) ;
#14688=CIRCLE ( 'NONE', #578, 0.5000000000000004441 ) ;
#14690=EDGE_CURVE ( 'NONE', #7288, #3704, #2253, .T. ) ;
#14694=DIRECTION ( 'NONE',  ( 0.000000000000000000, 4.956352788505162775E-17, -1.000000000000000000 ) ) ;
#14698=DIRECTION ( 'NONE',  ( 0.000000000000000000, 0.000000000000000000, 1.000000000000000000 ) ) ;
#14700=CYLINDRICAL_SURFACE ( 'NONE', #7836, 0.5000000000000004441 ) ;
#14702=FACE_OUTER_BOUND ( 'NONE', #6339, .T. ) ;
#14705=CARTESIAN_POINT ( 'NONE',  ( -70.00000000000000000, -201.3058001507315566, 77.95141194869098911 ) ) ;
#14706=CYLINDRICAL_SURFACE ( 'NONE', #9717, 0.4999999999999996114 ) ;
#14707=AXIS2_PLACEMENT_3D ( 'NONE', #8742, #1382, #6220 ) ;
#14718=EDGE_CURVE ( 'NONE', #14008, #830, #980, .T. ) ;
#14726=EDGE_CURVE ( 'NONE', #10971, #8310, #5522, .T. ) ;
#14730=EDGE_LOOP ( 'NONE', ( #10768, #22, #12332, #2258 ) ) ;
#14739=DIRECTION ( 'NONE',  ( -3.862829527358613429E-15, 0.9902680687415705840, -0.1391731009600641333 ) ) ;
#14740=FACE_OUTER_BOUND ( 'NONE', #2710, .T. ) ;
#14742=ORIENTED_EDGE ( 'NONE', *, *, #4402, .F. ) ;
#14743=ADVANCED_FACE ( 'NONE', ( #6368 ), #7550, .F. ) ;
#14746=VERTEX_POINT ( 'NONE', #9760 ) ;
#14752=VERTEX_POINT ( 'NONE', #12348 ) ;
#14754=DIRECTION ( 'NONE',  ( 0.000000000000000000, -1.000000000000000000, 0.000000000000000000 ) ) ;
#14755=TOROIDAL_SURFACE ( 'NONE', #893, 1.000000000000000000, 0.5000000000000000000 ) ;
#14757=DIRECTION ( 'NONE',  ( 0.000000000000000000, -0.9902680687415702510, 0.1391731009600660485 ) ) ;
#14759=ADVANCED_FACE ( 'NONE', ( #12191 ), #12074, .T. ) ;
#14765=VECTOR ( 'NONE', #5556, 1000.000000000000000 ) ;
#14766=DIRECTION ( 'NONE',  ( 0.000000000000000000, 4.956352788505162775E-17, -1.000000000000000000 ) ) ;
#14773=DIRECTION ( 'NONE',  ( -1.000000000000000000, 0.000000000000000000, 0.000000000000000000 ) ) ;
#14779=CARTESIAN_POINT ( 'NONE',  ( -64.00000000000002842, 15.03993994372673981, -3.075184203610571654 ) ) ;
#14786=VERTEX_POINT ( 'NONE', #7322 ) ;
#14788=EDGE_CURVE ( 'NONE', #620, #12158, #14327, .T. ) ;
#14802=ORIENTED_EDGE ( 'NONE', *, *, #10492, .F. ) ;
#14803=CARTESIAN_POINT ( 'NONE',  ( 178.0000000000000853, 14.97035339324670922, -2.580050169239785696 ) ) ;
#14804=FACE_OUTER_BOUND ( 'NONE', #10276, .T. ) ;
#14808=CARTESIAN_POINT ( 'NONE',  ( -63.50000000000002842, -178.8058001507315566, 65.31842631998698323 ) ) ;
#14809=DIRECTION ( 'NONE',  ( 0.000000000000000000, 1.000000000000000000, 6.938893903907227145E-17 ) ) ;
#14813=EDGE_CURVE ( 'NONE', #5911, #11697, #5764, .T. ) ;
#14816=CARTESIAN_POINT ( 'NONE',  ( 190.5000000000000568, 15.03993994372673981, -2.075184203610571210 ) ) ;
#14821=CARTESIAN_POINT ( 'NONE',  ( 190.5000000000000853, 17.53993994372673626, 52.49999999999997868 ) ) ;
#14823=ADVANCED_FACE ( 'NONE', ( #7471 ), #14638, .T. ) ;
#14827=CARTESIAN_POINT ( 'NONE',  ( 190.5000000000000853, 15.53993994372673626, 52.49999999999997868 ) ) ;
#14828=AXIS2_PLACEMENT_3D ( 'NONE', #9034, #14350, #3547 ) ;
#14829=CIRCLE ( 'NONE', #9806, 0.5000000000000004441 ) ;
#14831=ORIENTED_EDGE ( 'NONE', *, *, #4052, .T. ) ;
#14834=DIRECTION ( 'NONE',  ( -0.000000000000000000, 1.000000000000000000, 6.938893903907222067E-15 ) ) ;
#14835=AXIS2_PLACEMENT_3D ( 'NONE', #13198, #3587, #160 ) ;
#14838=PLANE ( 'NONE',  #3169 ) ;
#14839=TOROIDAL_SURFACE ( 'NONE', #718, 1.000000000000000000, 0.5000000000000000000 ) ;
#14843=EDGE_LOOP ( 'NONE', ( #5960, #14496, #279, #7883 ) ) ;
#14845=DIRECTION ( 'NONE',  ( 0.000000000000000000, 1.734723475976806306E-15, -1.000000000000000000 ) ) ;
#14848=ORIENTED_EDGE ( 'NONE', *, *, #13957, .F. ) ;
#14851=AXIS2_PLACEMENT_3D ( 'NONE', #12960, #2309, #2 ) ;
#14853=CARTESIAN_POINT ( 'NONE',  ( -63.50000000000002842, -178.7362136002515172, 52.68580191161573367 ) ) ;
#14854=AXIS2_PLACEMENT_3D ( 'NONE', #9873, #12070, #12294 ) ;
#14860=DIRECTION ( 'NONE',  ( 0.000000000000000000, -0.1391731009600592484, -0.9902680687415712502 ) ) ;
#14863=ORIENTED_EDGE ( 'NONE', *, *, #534, .F. ) ;
#14866=ORIENTED_EDGE ( 'NONE', *, *, #11033, .T. ) ;
#14867=CARTESIAN_POINT ( 'NONE',  ( 190.5000000000000568, 15.53993994372673981, -17.50000000000002487 ) ) ;
#14871=CARTESIAN_POINT ( 'NONE',  ( -76.50000000000004263, 15.53993994372673626, 52.49999999999997868 ) ) ;
#14873=AXIS2_PLACEMENT_3D ( 'NONE', #6066, #4791, #7181 ) ;
#14874=CARTESIAN_POINT ( 'NONE',  ( -76.00000000000004263, -179.8058001507315566, 65.31842631998698323 ) ) ;
#14875=ADVANCED_FACE ( 'NONE', ( #13524 ), #6027, .T. ) ;
#14879=CARTESIAN_POINT ( 'NONE',  ( -64.00000000000002842, -179.8058001507315566, 65.31842631998698323 ) ) ;
#14882=ORIENTED_EDGE ( 'NONE', *, *, #12225, .T. ) ;
#14883=VECTOR ( 'NONE', #15538, 1000.000000000000000 ) ;
#14888=DIRECTION ( 'NONE',  ( -1.000000000000000000, 0.000000000000000000, 0.000000000000000000 ) ) ;
#14892=CARTESIAN_POINT ( 'NONE',  ( 178.0000000000000853, -178.9449732516916072, 64.32815825124539799 ) ) ;
#14896=CARTESIAN_POINT ( 'NONE',  ( 190.5000000000000568, -179.3058001507315566, 52.19066787724494816 ) ) ;
#14904=ADVANCED_FACE ( 'NONE', ( #8971 ), #4510, .T. ) ;
#14907=DIRECTION ( 'NONE',  ( -0.000000000000000000, 1.000000000000000000, -0.000000000000000000 ) ) ;
#14909=ORIENTED_EDGE ( 'NONE', *, *, #445, .T. ) ;
#14912=EDGE_CURVE ( 'NONE', #6496, #8328, #14829, .T. ) ;
#14913=CIRCLE ( 'NONE', #789, 0.5000000000000004441 ) ;
#14915=ORIENTED_EDGE ( 'NONE', *, *, #13956, .F. ) ;
#14920=ORIENTED_EDGE ( 'NONE', *, *, #13262, .F. ) ;
#14921=CARTESIAN_POINT ( 'NONE',  ( 190.0000000000000853, 15.53993994372673804, 37.49999999999991473 ) ) ;
#14926=CARTESIAN_POINT ( 'NONE',  ( 177.5000000000000853, -179.8058001507315566, -17.76585208085566947 ) ) ;
#14930=CARTESIAN_POINT ( 'NONE',  ( -64.00000000000002842, -179.3058001507315566, 52.19066787724494816 ) ) ;
#14935=AXIS2_PLACEMENT_3D ( 'NONE', #3800, #8622, #8476 ) ;
#14936=EDGE_CURVE ( 'NONE', #8234, #10763, #8807, .T. ) ;
#14947=ORIENTED_EDGE ( 'NONE', *, *, #10504, .F. ) ;
#14949=DIRECTION ( 'NONE',  ( -1.000000000000000000, -0.000000000000000000, -0.000000000000000000 ) ) ;
#14951=VECTOR ( 'NONE', #12688, 1000.000000000000000 ) ;
#14953=ORIENTED_EDGE ( 'NONE', *, *, #2246, .F. ) ;
#14954=CYLINDRICAL_SURFACE ( 'NONE', #11223, 0.5000000000000004441 ) ;
#14959=CARTESIAN_POINT ( 'NONE',  ( 178.0000000000000853, 15.53993994372674159, -17.50000000000002487 ) ) ;
#14967=AXIS2_PLACEMENT_3D ( 'NONE', #1657, #11454, #616 ) ;
#14968=DIRECTION ( 'NONE',  ( -1.000000000000000000, -0.000000000000000000, -0.000000000000000000 ) ) ;
#14969=EDGE_LOOP ( 'NONE', ( #11050, #12771, #9684, #1576 ) ) ;
#14970=EDGE_CURVE ( 'NONE', #6505, #3793, #3115, .T. ) ;
#14971=CARTESIAN_POINT ( 'NONE',  ( -76.50000000000004263, 15.03993994372673804, 38.07518420361041933 ) ) ;
#14982=CARTESIAN_POINT ( 'NONE',  ( -63.50000000000002842, 15.53993994372673626, 52.49999999999997868 ) ) ;
#14983=DIRECTION ( 'NONE',  ( 5.518327896226373923E-17, 0.9902680687415712502, 0.1391731009600586100 ) ) ;
#14984=ADVANCED_FACE ( 'NONE', ( #9043 ), #11319, .T. ) ;
#14985=VECTOR ( 'NONE', #14166, 1000.000000000000000 ) ;
#14986=CARTESIAN_POINT ( 'NONE',  ( 177.5000000000000853, -178.8753867012115961, -29.82329228561640022 ) ) ;
#14988=EDGE_CURVE ( 'NONE', #13434, #8877, #10069, .T. ) ;
#14997=DIRECTION ( 'NONE',  ( 0.000000000000000000, -1.000000000000000000, -0.000000000000000000 ) ) ;
#15003=AXIS2_PLACEMENT_3D ( 'NONE', #3504, #11960, #8342 ) ;
#15004=DIRECTION ( 'NONE',  ( 1.000000000000000000, 0.000000000000000000, 0.000000000000000000 ) ) ;
#15008=CARTESIAN_POINT ( 'NONE',  ( -70.00000000000000000, 17.53993994372673981, -12.49999999999999289 ) ) ;
#15009=CARTESIAN_POINT ( 'NONE',  ( 184.0000000000000568, 17.53993994372673626, 48.99999999999997158 ) ) ;
#15010=DIRECTION ( 'NONE',  ( -1.000000000000000000, 0.000000000000000000, 0.000000000000000000 ) ) ;
#15014=EDGE_CURVE ( 'NONE', #9239, #8771, #14586, .T. ) ;
#15015=DIRECTION ( 'NONE',  ( 1.000000000000000000, -2.751328491981765035E-32, 3.965082230804130220E-16 ) ) ;
#15016=ORIENTED_EDGE ( 'NONE', *, *, #4772, .F. ) ;
#15024=AXIS2_PLACEMENT_3D ( 'NONE', #15449, #4648, #14427 ) ;
#15027=CARTESIAN_POINT ( 'NONE',  ( -63.50000000000002842, -179.8058001507315566, -17.76585208085566947 ) ) ;
#15029=DIRECTION ( 'NONE',  ( 0.000000000000000000, 1.000000000000000000, 0.000000000000000000 ) ) ;
#15033=CARTESIAN_POINT ( 'NONE',  ( -64.00000000000002842, 15.17911304468679745, 25.93769382960995529 ) ) ;
#15037=ORIENTED_EDGE ( 'NONE', *, *, #14372, .F. ) ;
#15040=DIRECTION ( 'NONE',  ( 1.000000000000000000, 2.751328491981765035E-32, -3.965082230804130220E-16 ) ) ;
#15041=CARTESIAN_POINT ( 'NONE',  ( 178.0000000000000853, 16.03993994372673981, -17.50000000000002487 ) ) ;
#15045=CARTESIAN_POINT ( 'NONE',  ( -76.00000000000001421, -179.3058001507315566, -17.76585208085566947 ) ) ;
#15046=DIRECTION ( 'NONE',  ( 5.518327896226364679E-17, -0.9902680687415713612, 0.1391731009600582492 ) ) ;
#15050=EDGE_CURVE ( 'NONE', #4447, #7175, #6910, .T. ) ;
#15054=EDGE_LOOP ( 'NONE', ( #14375, #8776, #11139, #15175 ) ) ;
#15055=ADVANCED_FACE ( 'NONE', ( #6834 ), #7146, .F. ) ;
#15059=FACE_OUTER_BOUND ( 'NONE', #6184, .T. ) ;
#15060=DIRECTION ( 'NONE',  ( -0.000000000000000000, 1.000000000000000000, 6.938893903907227145E-17 ) ) ;
#15064=ADVANCED_FACE ( 'NONE', ( #4677 ), #14839, .T. ) ;
#15066=CIRCLE ( 'NONE', #695, 1.499999999999994449 ) ;
#15068=ORIENTED_EDGE ( 'NONE', *, *, #15288, .T. ) ;
#15073=DIRECTION ( 'NONE',  ( -3.965082230804130220E-16, -0.000000000000000000, -1.000000000000000000 ) ) ;
#15078=DIRECTION ( 'NONE',  ( 1.000000000000000000, 0.000000000000000000, 0.000000000000000000 ) ) ;
#15086=DIRECTION ( 'NONE',  ( -0.000000000000000000, -0.000000000000000000, 1.000000000000000000 ) ) ;
#15089=FACE_OUTER_BOUND ( 'NONE', #13777, .T. ) ;
#15090=EDGE_LOOP ( 'NONE', ( #10514, #9756, #4344, #6721 ) ) ;
#15093=DIRECTION ( 'NONE',  ( -3.965082230804130220E-16, 1.090924371466202084E-47, 1.000000000000000000 ) ) ;
#15094=ORIENTED_EDGE ( 'NONE', *, *, #3586, .T. ) ;
#15098=ORIENTED_EDGE ( 'NONE', *, *, #12028, .F. ) ;
#15099=ADVANCED_FACE ( 'NONE', ( #4366 ), #11721, .F. ) ;
#15102=CIRCLE ( 'NONE', #9567, 0.5000000000000000000 ) ;
#15103=DIRECTION ( 'NONE',  ( -0.000000000000000000, -0.9902680687415711391, -0.1391731009600593039 ) ) ;
#15106=AXIS2_PLACEMENT_3D ( 'NONE', #13220, #4707, #15430 ) ;
#15119=CARTESIAN_POINT ( 'NONE',  ( -70.00000000000000000, -179.3058001507315566, 76.45141194869098911 ) ) ;
#15121=VECTOR ( 'NONE', #4241, 1000.000000000000000 ) ;
#15151=DIRECTION ( 'NONE',  ( 1.000000000000000000, 0.000000000000000000, 0.000000000000000000 ) ) ;
#15152=TOROIDAL_SURFACE ( 'NONE', #5087, 1.000000000000000000, 0.5000000000000000000 ) ;
#15155=VERTEX_POINT ( 'NONE', #13032 ) ;
#15165=AXIS2_PLACEMENT_3D ( 'NONE', #11035, #3771, #187 ) ;
#15169=DIRECTION ( 'NONE',  ( -1.000000000000000000, 0.000000000000000000, 0.000000000000000000 ) ) ;
#15175=ORIENTED_EDGE ( 'NONE', *, *, #1390, .T. ) ;
#15179=LINE ( 'NONE', #12815, #14508 ) ;
#15181=CARTESIAN_POINT ( 'NONE',  ( 190.5000000000000568, 16.03993994372673981, 10.05257423913146475 ) ) ;
#15183=DIRECTION ( 'NONE',  ( -3.965082230804130220E-16, 1.090924371466202084E-47, 1.000000000000000000 ) ) ;
#15184=ADVANCED_FACE ( 'NONE', ( #2154 ), #962, .T. ) ;
#15185=ADVANCED_FACE ( 'NONE', ( #15247 ), #4442, .F. ) ;
#15193=VERTEX_POINT ( 'NONE', #12174 ) ;
#15194=CARTESIAN_POINT ( 'NONE',  ( -76.50000000000004263, -178.8058001507315566, 52.19066787724494816 ) ) ;
#15196=ORIENTED_EDGE ( 'NONE', *, *, #7340, .F. ) ;
#15198=CYLINDRICAL_SURFACE ( 'NONE', #15366, 0.5000000000000004441 ) ;
#15200=DIRECTION ( 'NONE',  ( 0.000000000000000000, 0.000000000000000000, -1.000000000000000000 ) ) ;
#15204=DIRECTION ( 'NONE',  ( -1.000000000000000000, -0.000000000000000000, -0.000000000000000000 ) ) ;
#15205=EDGE_CURVE ( 'NONE', #10763, #4290, #2393, .T. ) ;
#15206=CIRCLE ( 'NONE', #10439, 1.000000000000000888 ) ;
#15212=VERTEX_POINT ( 'NONE', #3890 ) ;
#15216=CARTESIAN_POINT ( 'NONE',  ( 178.0000000000000853, 15.03993994372673804, 24.94742576086838781 ) ) ;
#15220=LINE ( 'NONE', #10581, #3802 ) ;
#15221=ADVANCED_FACE ( 'NONE', ( #9900 ), #4845, .F. ) ;
#15223=ORIENTED_EDGE ( 'NONE', *, *, #13565, .F. ) ;
#15225=ORIENTED_EDGE ( 'NONE', *, *, #9721, .F. ) ;
#15228=ORIENTED_EDGE ( 'NONE', *, *, #10764, .T. ) ;
#15230=ORIENTED_EDGE ( 'NONE', *, *, #12782, .T. ) ;
#15232=DIRECTION ( 'NONE',  ( 2.751328491981765035E-32, 1.000000000000000000, 1.090924371466202084E-47 ) ) ;
#15233=CARTESIAN_POINT ( 'NONE',  ( 178.0000000000000853, -179.3058001507315566, 84.88378295107887084 ) ) ;
#15234=CIRCLE ( 'NONE', #7955, 0.5000000000000004441 ) ;
#15235=VERTEX_POINT ( 'NONE', #7300 ) ;
#15241=DIRECTION ( 'NONE',  ( 0.000000000000000000, 0.000000000000000000, -1.000000000000000000 ) ) ;
#15244=FACE_OUTER_BOUND ( 'NONE', #5652, .T. ) ;
#15247=FACE_OUTER_BOUND ( 'NONE', #3402, .T. ) ;
#15255=CIRCLE ( 'NONE', #3679, 1.000000000000000888 ) ;
#15256=DIRECTION ( 'NONE',  ( 0.000000000000000000, -6.938893903907227145E-17, 1.000000000000000000 ) ) ;
#15259=DIRECTION ( 'NONE',  ( 1.000000000000000000, 0.000000000000000000, 0.000000000000000000 ) ) ;
#15264=CARTESIAN_POINT ( 'NONE',  ( -64.00000000000002842, -179.8058001507315566, 52.49999999999997868 ) ) ;
#15266=AXIS2_PLACEMENT_3D ( 'NONE', #9116, #4275, #12563 ) ;
#15269=ORIENTED_EDGE ( 'NONE', *, *, #1267, .F. ) ;
#15270=ORIENTED_EDGE ( 'NONE', *, *, #335, .T. ) ;
#15272=DIRECTION ( 'NONE',  ( 0.000000000000000000, 0.1391731009600626345, 0.9902680687415706950 ) ) ;
#15274=CARTESIAN_POINT ( 'NONE',  ( -63.50000000000002842, 16.03993994372673626, 38.07518420361041933 ) ) ;
#15279=PRODUCT_DEFINITION_CONTEXT ( 'detailed design', #10193, 'design' ) ;
#15280=DIRECTION ( 'NONE',  ( -1.000000000000000000, -0.000000000000000000, -0.000000000000000000 ) ) ;
#15286=CARTESIAN_POINT ( 'NONE',  ( 190.0000000000000853, 15.10952649420676686, 25.44255979523916977 ) ) ;
#15288=EDGE_CURVE ( 'NONE', #6079, #1572, #4010, .T. ) ;
#15292=DIRECTION ( 'NONE',  ( 0.000000000000000000, 0.000000000000000000, -1.000000000000000000 ) ) ;
#15297=ORIENTED_EDGE ( 'NONE', *, *, #10235, .F. ) ;
#15299=LINE ( 'NONE', #939, #2827 ) ;
#15300=ORIENTED_EDGE ( 'NONE', *, *, #4911, .F. ) ;
#15302=CARTESIAN_POINT ( 'NONE',  ( -76.50000000000004263, 15.53993994372673626, 52.49999999999997868 ) ) ;
#15304=FACE_BOUND ( 'NONE', #4265, .T. ) ;
#15306=VERTEX_POINT ( 'NONE', #8414 ) ;
#15309=EDGE_LOOP ( 'NONE', ( #7375, #5682, #12250, #2691 ) ) ;
#15310=AXIS2_PLACEMENT_3D ( 'NONE', #15041, #13788, #2023 ) ;
#15316=CIRCLE ( 'NONE', #8544, 1.499999999999994449 ) ;
#15323=CARTESIAN_POINT ( 'NONE',  ( -70.00000000000000000, -201.3058001507315566, -39.95141194869120937 ) ) ;
#15325=ORIENTED_EDGE ( 'NONE', *, *, #2663, .F. ) ;
#15330=CARTESIAN_POINT ( 'NONE',  ( -76.00000000000001421, 11.87216911405867670, 8.597545510065431884 ) ) ;
#15331=VECTOR ( 'NONE', #9392, 1000.000000000000000 ) ;
#15332=DIRECTION ( 'NONE',  ( -1.000000000000000000, -2.751328491981765035E-32, 3.965082230804130220E-16 ) ) ;
#15333=AXIS2_PLACEMENT_3D ( 'NONE', #9999, #4865, #10872 ) ;
#15334=ORIENTED_EDGE ( 'NONE', *, *, #13550, .F. ) ;
#15335=DIRECTION ( 'NONE',  ( 0.000000000000000000, 0.000000000000000000, -1.000000000000000000 ) ) ;
#15336=EDGE_CURVE ( 'NONE', #11925, #6214, #10075, .T. ) ;
#15338=ORIENTED_EDGE ( 'NONE', *, *, #9467, .T. ) ;
#15339=CYLINDRICAL_SURFACE ( 'NONE', #1365, 1.500000000000001332 ) ;
#15344=DIRECTION ( 'NONE',  ( -0.000000000000000000, -0.000000000000000000, -1.000000000000000000 ) ) ;
#15345=ORIENTED_EDGE ( 'NONE', *, *, #164, .T. ) ;
#15347=CARTESIAN_POINT ( 'NONE',  ( 190.5000000000000568, -179.3058001507315566, 84.88378295107887084 ) ) ;
#15348=DIRECTION ( 'NONE',  ( -3.965082230804130220E-16, 4.956352788505162775E-17, -1.000000000000000000 ) ) ;
#15353=AXIS2_PLACEMENT_3D ( 'NONE', #7061, #879, #9423 ) ;
#15357=DIRECTION ( 'NONE',  ( 1.000000000000000000, -2.751328491981765035E-32, 3.965082230804130220E-16 ) ) ;
#15359=DIRECTION ( 'NONE',  ( 0.000000000000000000, -0.1391731009600591096, 0.9902680687415711391 ) ) ;
#15366=AXIS2_PLACEMENT_3D ( 'NONE', #12918, #4551, #8046 ) ;
#15376=ORIENTED_EDGE ( 'NONE', *, *, #11267, .T. ) ;
#15377=CIRCLE ( 'NONE', #6592, 0.5000000000000004441 ) ;
#15381=EDGE_CURVE ( 'NONE', #3488, #9726, #10049, .T. ) ;
#15382=EDGE_CURVE ( 'NONE', #3829, #10747, #3020, .T. ) ;
#15384=EDGE_LOOP ( 'NONE', ( #13898, #5614, #8540, #6803 ) ) ;
#15386=DIRECTION ( 'NONE',  ( 1.000000000000000000, 0.000000000000000000, 0.000000000000000000 ) ) ;
#15388=EDGE_CURVE ( 'NONE', #12671, #13452, #10583, .T. ) ;
#15389=ORIENTED_EDGE ( 'NONE', *, *, #9891, .F. ) ;
#15390=CYLINDRICAL_SURFACE ( 'NONE', #3741, 0.5000000000000004441 ) ;
#15392=VECTOR ( 'NONE', #1904, 1000.000000000000000 ) ;
#15394=DIRECTION ( 'NONE',  ( 0.000000000000000000, 0.1391731009600660485, -0.9902680687415702510 ) ) ;
#15395=DIRECTION ( 'NONE',  ( 1.000000000000000000, 0.000000000000000000, 0.000000000000000000 ) ) ;
#15397=ORIENTED_EDGE ( 'NONE', *, *, #6049, .T. ) ;
#15398=EDGE_CURVE ( 'NONE', #2407, #815, #2945, .T. ) ;
#15399=CARTESIAN_POINT ( 'NONE',  ( -76.00000000000004263, -179.3058001507316419, 52.76585208085545986 ) ) ;
#15402=DIRECTION ( 'NONE',  ( 1.000000000000000000, 0.000000000000000000, 0.000000000000000000 ) ) ;
#15404=DIRECTION ( 'NONE',  ( 1.000000000000000000, 0.000000000000000000, 0.000000000000000000 ) ) ;
#15405=ORIENTED_EDGE ( 'NONE', *, *, #8548, .T. ) ;
#15417=ADVANCED_BREP_SHAPE_REPRESENTATION ( '', ( #5438, #10819, #12337 ), #180 ) ;
#15426=CARTESIAN_POINT ( 'NONE',  ( -76.50000000000004263, -179.8058001507315566, 52.76585208085545275 ) ) ;
#15429=CARTESIAN_POINT ( 'NONE',  ( 190.0000000000000568, 15.17911304468679923, 9.062306170389897275 ) ) ;
#15430=DIRECTION ( 'NONE',  ( 0.000000000000000000, -1.000000000000000000, -6.938893903907227145E-17 ) ) ;
#15431=CYLINDRICAL_SURFACE ( 'NONE', #73, 0.4999999999999996114 ) ;
#15434=ADVANCED_FACE ( 'NONE', ( #7613, #12407 ), #1591, .F. ) ;
#15436=VECTOR ( 'NONE', #14888, 1000.000000000000000 ) ;
#15440=CARTESIAN_POINT ( 'NONE',  ( 190.0000000000000568, 15.03993994372673804, 24.94742576086838781 ) ) ;
#15442=ORIENTED_EDGE ( 'NONE', *, *, #2656, .F. ) ;
#15444=CARTESIAN_POINT ( 'NONE',  ( -76.00000000000004263, -179.8058001507315566, 84.88378295107887084 ) ) ;
#15446=AXIS2_PLACEMENT_3D ( 'NONE', #14102, #7973, #4236 ) ;
#15449=CARTESIAN_POINT ( 'NONE',  ( 184.0000000000000568, -181.3058001507315566, 76.45141194869098911 ) ) ;
#15454=ORIENTED_EDGE ( 'NONE', *, *, #9952, .T. ) ;
#15459=CARTESIAN_POINT ( 'NONE',  ( 190.0000000000000568, -179.8058001507315566, -17.50000000000002487 ) ) ;
#15463=PLANE ( 'NONE',  #7345 ) ;
#15464=DIRECTION ( 'NONE',  ( -0.000000000000000000, -0.000000000000000000, 1.000000000000000000 ) ) ;
#15467=DIRECTION ( 'NONE',  ( 0.000000000000000000, 4.956352788505162775E-17, -1.000000000000000000 ) ) ;
#15469=DIRECTION ( 'NONE',  ( 0.000000000000000000, 0.000000000000000000, -1.000000000000000000 ) ) ;
#15473=CIRCLE ( 'NONE', #1357, 1.000000000000000888 ) ;
#15474=EDGE_CURVE ( 'NONE', #10070, #2702, #952, .T. ) ;
#15475=CARTESIAN_POINT ( 'NONE',  ( 184.0000000000000568, -181.3058001507315566, -39.95141194869120937 ) ) ;
#15477=ORIENTED_EDGE ( 'NONE', *, *, #10664, .F. ) ;
#15483=VERTEX_POINT ( 'NONE', #9337 ) ;
#15486=ORIENTED_EDGE ( 'NONE', *, *, #5460, .T. ) ;
#15488=LINE ( 'NONE', #4685, #4779 ) ;
#15490=ADVANCED_FACE ( 'NONE', ( #15304, #4348 ), #943, .T. ) ;
#15497=ORIENTED_EDGE ( 'NONE', *, *, #823, .F. ) ;
#15501=CARTESIAN_POINT ( 'NONE',  ( 178.0000000000000853, 14.90076684276667862, 37.08491613486885541 ) ) ;
#15503=EDGE_CURVE ( 'NONE', #8234, #12311, #9791, .T. ) ;
#15509=AXIS2_PLACEMENT_3D ( 'NONE', #15330, #3431, #8263 ) ;
#15510=DIRECTION ( 'NONE',  ( -1.000000000000000000, 0.000000000000000000, 0.000000000000000000 ) ) ;
#15511=CARTESIAN_POINT ( 'NONE',  ( 178.0000000000000853, 15.53993994372673804, 37.49999999999991473 ) ) ;
#15518=EDGE_CURVE ( 'NONE', #12077, #1137, #5545, .T. ) ;
#15522=ORIENTED_EDGE ( 'NONE', *, *, #6824, .F. ) ;
#15524=CARTESIAN_POINT ( 'NONE',  ( -70.00000000000000000, 15.53993994372673626, 45.99999999999998579 ) ) ;
#15531=DIRECTION ( 'NONE',  ( 0.000000000000000000, 0.1391731009600591096, -0.9902680687415711391 ) ) ;
#15536=ORIENTED_EDGE ( 'NONE', *, *, #13204, .F. ) ;
#15537=DIRECTION ( 'NONE',  ( -0.000000000000000000, 1.000000000000000000, -0.000000000000000000 ) ) ;
#15538=DIRECTION ( 'NONE',  ( 3.965082230804130220E-16, 4.956352788505162775E-17, -1.000000000000000000 ) ) ;
#15539=ORIENTED_EDGE ( 'NONE', *, *, #9049, .T. ) ;
#15551=AXIS2_PLACEMENT_3D ( 'NONE', #4512, #9344, #14140 ) ;
#15553=DIRECTION ( 'NONE',  ( 0.000000000000000000, 1.000000000000000000, 0.000000000000000000 ) ) ;
#15554=ORIENTED_EDGE ( 'NONE', *, *, #4830, .F. ) ;
#15555=EDGE_LOOP ( 'NONE', ( #14848, #10136, #3865, #862 ) ) ;
#15559=ORIENTED_EDGE ( 'NONE', *, *, #10533, .T. ) ;
#15562=DIRECTION ( 'NONE',  ( -0.000000000000000000, -4.956352788505162775E-17, 1.000000000000000000 ) ) ;
#15565=AXIS2_PLACEMENT_3D ( 'NONE', #14879, #4222, #2905 ) ;
#15572=EDGE_CURVE ( 'NONE', #2689, #12589, #9541, .T. ) ;
#15574=CARTESIAN_POINT ( 'NONE',  ( -76.50000000000001421, 15.10952649420676686, 25.44255979523916977 ) ) ;
#15581=ORIENTED_EDGE ( 'NONE', *, *, #5761, .T. ) ;
#15587=CARTESIAN_POINT ( 'NONE',  ( -76.50000000000004263, 15.17911304468679745, 25.93769382960994818 ) ) ;
#15592=VECTOR ( 'NONE', #8541, 1000.000000000000000 ) ;
#15594=CARTESIAN_POINT ( 'NONE',  ( -63.50000000000002842, 17.53993994372673981, -17.50000000000002487 ) ) ;
#15595=VECTOR ( 'NONE', #5945, 1000.000000000000000 ) ;
#15602=CIRCLE ( 'NONE', #9085, 1.000000000000000888 ) ;
#15603=DIRECTION ( 'NONE',  ( 0.000000000000000000, 1.000000000000000000, 0.000000000000000000 ) ) ;
#15606=( NAMED_UNIT ( * ) PLANE_ANGLE_UNIT ( ) SI_UNIT ( $, .RADIAN. ) );
#15610=DIRECTION ( 'NONE',  ( 0.000000000000000000, 0.000000000000000000, -1.000000000000000000 ) ) ;
#15614=AXIS2_PLACEMENT_3D ( 'NONE', #15264, #14246, #3290 ) ;
#15618=DIRECTION ( 'NONE',  ( 0.000000000000000000, 1.000000000000000000, 0.000000000000000000 ) ) ;
ENDSEC;
END-ISO-10303-21;
